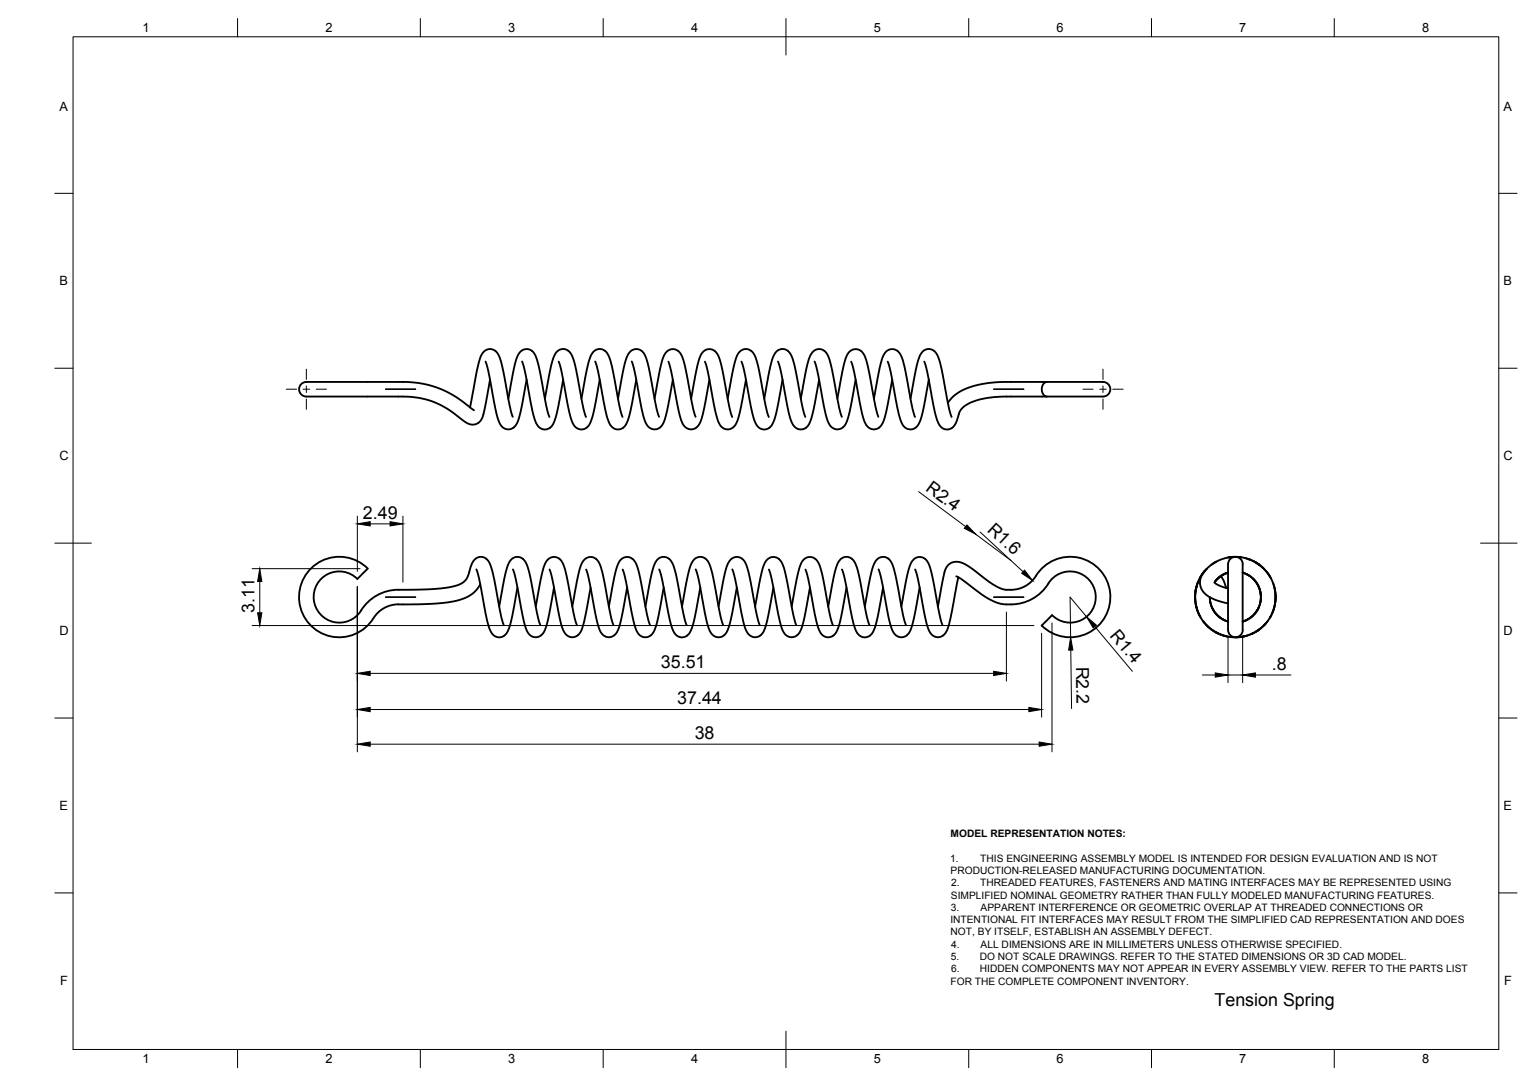
ISO-10303-21;
HEADER;
/* Generated by software containing ST-Developer
 * from STEP Tools, Inc. (www.steptools.com) 
 */

FILE_DESCRIPTION(
/* description */ ('STEP AP214'),
/* implementation_level */ '2;1');

FILE_NAME(
/* name */ 'Tension Spring.step',
/* time_stamp */ '2026-10-06T11:11:25-07:00',
/* author */ (''),
/* organization */ (''),
/* preprocessor_version */ 'ST-DEVELOPER v20.2',
/* originating_system */ 'Autodesk Translation Framework v15.15.0.0',
/* authorisation */ '');

FILE_SCHEMA (('AUTOMOTIVE_DESIGN { 1 0 10303 214 3 1 1 }'));
ENDSEC;

DATA;
#10=MECHANICAL_DESIGN_GEOMETRIC_PRESENTATION_REPRESENTATION('',(#699),#47717);
#148=B_SPLINE_CURVE_WITH_KNOTS('',3,(#12437,#12438,#12439,#12440,#12441,
#12442,#12443,#12444,#12445,#12446,#12447,#12448,#12449,#12450,#12451,#12452,
#12453,#12454,#12455,#12456,#12457,#12458,#12459,#12460),.UNSPECIFIED.,
 .F.,.F.,(4,2,2,2,2,2,2,2,2,2,2,4),(0.916063809045508,0.917441355582055,
0.918818902118601,0.921573995191693,0.924329088264786,0.925706634801332,
0.927084181337879,0.932594367484064,0.935349460557156,0.936727007093702,
0.937415780361976,0.938104553630249),.UNSPECIFIED.);
#149=B_SPLINE_CURVE_WITH_KNOTS('',3,(#12461,#12462,#12463,#12464,#12465,
#12466,#12467,#12468,#12469,#12470,#12471,#12472,#12473,#12474,#12475,#12476,
#12477,#12478,#12479,#12480,#12481,#12482,#12483,#12484),.UNSPECIFIED.,
 .F.,.F.,(4,2,2,2,2,2,2,2,2,2,2,4),(0.916063809045508,0.917441355582055,
0.918818902118601,0.921573995191693,0.924329088264786,0.925706634801332,
0.927084181337879,0.932594367484064,0.935349460557156,0.936727007093702,
0.937415780361976,0.938104553630249),.UNSPECIFIED.);
#150=B_SPLINE_CURVE_WITH_KNOTS('',3,(#13664,#13665,#13666,#13667,#13668,
#13669,#13670,#13671,#13672,#13673,#13674,#13675,#13676,#13677,#13678,#13679,
#13680,#13681,#13682,#13683,#13684,#13685,#13686,#13687,#13688,#13689,#13690,
#13691,#13692,#13693,#13694,#13695,#13696,#13697,#13698,#13699,#13700,#13701,
#13702,#13703,#13704,#13705,#13706,#13707,#13708,#13709,#13710,#13711,#13712,
#13713,#13714,#13715,#13716,#13717,#13718,#13719,#13720,#13721,#13722,#13723,
#13724,#13725,#13726,#13727,#13728,#13729,#13730,#13731,#13732,#13733,#13734,
#13735,#13736,#13737,#13738,#13739,#13740,#13741,#13742,#13743,#13744,#13745,
#13746,#13747,#13748,#13749,#13750,#13751,#13752,#13753,#13754,#13755,#13756,
#13757,#13758,#13759,#13760,#13761,#13762,#13763,#13764,#13765,#13766,#13767,
#13768,#13769,#13770,#13771,#13772,#13773,#13774,#13775,#13776,#13777,#13778,
#13779,#13780,#13781,#13782,#13783,#13784,#13785,#13786,#13787,#13788,#13789,
#13790,#13791,#13792,#13793,#13794,#13795,#13796,#13797,#13798,#13799,#13800,
#13801,#13802,#13803,#13804,#13805,#13806,#13807,#13808,#13809,#13810,#13811,
#13812,#13813,#13814,#13815,#13816,#13817,#13818,#13819,#13820,#13821,#13822,
#13823,#13824,#13825,#13826,#13827,#13828,#13829,#13830,#13831),
 .UNSPECIFIED.,.F.,.F.,(4,2,2,2,2,2,2,2,2,2,2,2,2,2,2,2,2,2,2,2,2,2,2,2,
2,2,2,2,2,2,2,2,2,2,2,2,2,2,2,2,2,2,2,2,2,2,2,2,2,2,2,2,2,2,2,2,2,2,2,2,
2,2,2,2,2,2,2,2,2,2,2,2,2,2,2,2,2,2,2,2,2,2,2,4),(0.0896131586159842,0.0909349273058256,
0.092256695995667,0.09490023337535,0.100187308134716,0.110761457653447,
0.121335607172179,0.131909756690911,0.142406945548381,0.152904134405852,
0.163401323263323,0.173898512120793,0.184326267064866,0.194754022008939,
0.205181776953011,0.215609531897084,0.225968774255778,0.236328016614473,
0.246687258973167,0.257046501331861,0.268365392558388,0.279684283784914,
0.29100317501144,0.302322066237966,0.313563979866736,0.324805893495506,
0.336047807124276,0.347289720753047,0.358457560536344,0.369625400319641,
0.380793240102939,0.391961079886236,0.403057648451734,0.414154217017233,
0.425250785582731,0.43634735414823,0.447375242283774,0.458403130419317,
0.469431018554861,0.480458906690405,0.491420626849432,0.50238234700846,
0.513344067167488,0.524305787326516,0.535203741266554,0.546101695206592,
0.55699964914663,0.567897603086667,0.578734005374906,0.589570407663145,
0.600406809951383,0.611243212239622,0.62202044333232,0.632797674425018,
0.643574905517716,0.654352136610414,0.665072195325672,0.675792254040929,
0.686512312756186,0.697232371471444,0.707897173370898,0.718561975270352,
0.729226777169807,0.739891579069261,0.750503305564763,0.761115032060264,
0.771726758555766,0.782338485051268,0.79289871583597,0.803458946620673,
0.814019177405375,0.824579408190078,0.835090233536042,0.845601058882007,
0.856111884227971,0.866622709573936,0.877085607262584,0.887548504951232,
0.89801140263988,0.908474300328528,0.912269054687018,0.914166431866263,
0.915115120455886,0.916063809045508),.UNSPECIFIED.);
#151=B_SPLINE_CURVE_WITH_KNOTS('',3,(#13832,#13833,#13834,#13835,#13836,
#13837,#13838,#13839,#13840,#13841,#13842,#13843,#13844,#13845,#13846,#13847,
#13848,#13849,#13850,#13851,#13852,#13853,#13854,#13855,#13856,#13857,#13858,
#13859,#13860,#13861,#13862,#13863,#13864,#13865,#13866,#13867,#13868,#13869,
#13870,#13871,#13872,#13873,#13874,#13875,#13876,#13877,#13878,#13879,#13880,
#13881,#13882,#13883,#13884,#13885,#13886,#13887,#13888,#13889,#13890,#13891,
#13892,#13893,#13894,#13895,#13896,#13897,#13898,#13899,#13900,#13901,#13902,
#13903,#13904,#13905,#13906,#13907,#13908,#13909,#13910,#13911,#13912,#13913,
#13914,#13915,#13916,#13917,#13918,#13919,#13920,#13921,#13922,#13923,#13924,
#13925,#13926,#13927,#13928,#13929,#13930,#13931,#13932,#13933,#13934,#13935,
#13936,#13937,#13938,#13939,#13940,#13941,#13942,#13943,#13944,#13945,#13946,
#13947,#13948,#13949,#13950,#13951,#13952,#13953,#13954,#13955,#13956,#13957,
#13958,#13959,#13960,#13961,#13962,#13963,#13964,#13965,#13966,#13967,#13968,
#13969,#13970,#13971,#13972,#13973,#13974,#13975,#13976,#13977,#13978,#13979,
#13980,#13981,#13982,#13983,#13984,#13985,#13986,#13987,#13988,#13989,#13990,
#13991,#13992,#13993,#13994,#13995,#13996,#13997,#13998,#13999),
 .UNSPECIFIED.,.F.,.F.,(4,2,2,2,2,2,2,2,2,2,2,2,2,2,2,2,2,2,2,2,2,2,2,2,
2,2,2,2,2,2,2,2,2,2,2,2,2,2,2,2,2,2,2,2,2,2,2,2,2,2,2,2,2,2,2,2,2,2,2,2,
2,2,2,2,2,2,2,2,2,2,2,2,2,2,2,2,2,2,2,2,2,2,2,4),(0.0896131586159842,0.0909349273058256,
0.092256695995667,0.09490023337535,0.100187308134716,0.110761457653447,
0.121335607172179,0.131909756690911,0.142406945548381,0.152904134405852,
0.163401323263323,0.173898512120793,0.184326267064866,0.194754022008939,
0.205181776953011,0.215609531897084,0.225968774255778,0.236328016614473,
0.246687258973167,0.257046501331861,0.268365392558388,0.279684283784914,
0.29100317501144,0.302322066237966,0.313563979866736,0.324805893495506,
0.336047807124276,0.347289720753047,0.358457560536344,0.369625400319641,
0.380793240102939,0.391961079886236,0.403057648451734,0.414154217017233,
0.425250785582731,0.43634735414823,0.447375242283774,0.458403130419317,
0.469431018554861,0.480458906690405,0.491420626849432,0.50238234700846,
0.513344067167488,0.524305787326516,0.535203741266554,0.546101695206592,
0.55699964914663,0.567897603086667,0.578734005374906,0.589570407663145,
0.600406809951383,0.611243212239622,0.62202044333232,0.632797674425018,
0.643574905517716,0.654352136610414,0.665072195325672,0.675792254040929,
0.686512312756186,0.697232371471444,0.707897173370898,0.718561975270352,
0.729226777169807,0.739891579069261,0.750503305564763,0.761115032060264,
0.771726758555766,0.782338485051268,0.79289871583597,0.803458946620673,
0.814019177405375,0.824579408190078,0.835090233536042,0.845601058882007,
0.856111884227971,0.866622709573936,0.877085607262584,0.887548504951232,
0.89801140263988,0.908474300328528,0.912269054687018,0.914166431866263,
0.915115120455886,0.916063809045508),.UNSPECIFIED.);
#152=B_SPLINE_CURVE_WITH_KNOTS('',3,(#14143,#14144,#14145,#14146,#14147,
#14148,#14149,#14150,#14151,#14152,#14153,#14154,#14155,#14156,#14157,#14158,
#14159,#14160,#14161,#14162),.UNSPECIFIED.,.F.,.F.,(4,2,2,2,2,2,2,2,2,4),
(0.0618954463697512,0.0653601604005303,0.0688248744313094,0.0757543024928677,
0.0792190165236468,0.0809513735390363,0.0826837305544259,0.086148444585205,
0.0878808016005946,0.0896131586159842),.UNSPECIFIED.);
#153=B_SPLINE_CURVE_WITH_KNOTS('',3,(#14163,#14164,#14165,#14166,#14167,
#14168,#14169,#14170,#14171,#14172,#14173,#14174,#14175,#14176,#14177,#14178,
#14179,#14180,#14181,#14182),.UNSPECIFIED.,.F.,.F.,(4,2,2,2,2,2,2,2,2,4),
(0.0618954463697512,0.0653601604005303,0.0688248744313094,0.0757543024928677,
0.0792190165236468,0.0809513735390363,0.0826837305544259,0.086148444585205,
0.0878808016005946,0.0896131586159842),.UNSPECIFIED.);
#526=(
BOUNDED_SURFACE()
B_SPLINE_SURFACE(3,3,((#12266,#12267,#12268,#12269,#12270,#12271,#12272,
#12273,#12274,#12275,#12276,#12277,#12278,#12279,#12280,#12281,#12282,#12283,
#12284,#12285,#12286,#12287,#12288,#12289),(#12290,#12291,#12292,#12293,
#12294,#12295,#12296,#12297,#12298,#12299,#12300,#12301,#12302,#12303,#12304,
#12305,#12306,#12307,#12308,#12309,#12310,#12311,#12312,#12313),(#12314,
#12315,#12316,#12317,#12318,#12319,#12320,#12321,#12322,#12323,#12324,#12325,
#12326,#12327,#12328,#12329,#12330,#12331,#12332,#12333,#12334,#12335,#12336,
#12337),(#12338,#12339,#12340,#12341,#12342,#12343,#12344,#12345,#12346,
#12347,#12348,#12349,#12350,#12351,#12352,#12353,#12354,#12355,#12356,#12357,
#12358,#12359,#12360,#12361),(#12362,#12363,#12364,#12365,#12366,#12367,
#12368,#12369,#12370,#12371,#12372,#12373,#12374,#12375,#12376,#12377,#12378,
#12379,#12380,#12381,#12382,#12383,#12384,#12385),(#12386,#12387,#12388,
#12389,#12390,#12391,#12392,#12393,#12394,#12395,#12396,#12397,#12398,#12399,
#12400,#12401,#12402,#12403,#12404,#12405,#12406,#12407,#12408,#12409),
(#12410,#12411,#12412,#12413,#12414,#12415,#12416,#12417,#12418,#12419,
#12420,#12421,#12422,#12423,#12424,#12425,#12426,#12427,#12428,#12429,#12430,
#12431,#12432,#12433)),.UNSPECIFIED.,.T.,.F.,.F.)
B_SPLINE_SURFACE_WITH_KNOTS((4,3,4),(4,2,2,2,2,2,2,2,2,2,2,4),(0.,0.5,1.),
(0.916063809045508,0.917441355582055,0.918818902118601,0.921573995191693,
0.924329088264786,0.925706634801332,0.927084181337879,0.932594367484064,
0.935349460557156,0.936727007093702,0.937415780361976,0.938104553630249),
 .UNSPECIFIED.)
GEOMETRIC_REPRESENTATION_ITEM()
RATIONAL_B_SPLINE_SURFACE(((1.,1.,1.,1.,1.,1.,1.,1.,1.,1.,1.,1.,1.,1.,1.,
1.,1.,1.,1.,1.,1.,1.,1.,1.),(0.333333333333333,0.333333333333333,0.333333333333333,
0.333333333333333,0.333333333333333,0.333333333333333,0.333333333333333,
0.333333333333333,0.333333333333333,0.333333333333333,0.333333333333333,
0.333333333333333,0.333333333333333,0.333333333333333,0.333333333333333,
0.333333333333333,0.333333333333333,0.333333333333333,0.333333333333333,
0.333333333333333,0.333333333333333,0.333333333333333,0.333333333333333,
0.333333333333333),(0.333333333333333,0.333333333333333,0.333333333333333,
0.333333333333333,0.333333333333333,0.333333333333333,0.333333333333333,
0.333333333333333,0.333333333333333,0.333333333333333,0.333333333333333,
0.333333333333333,0.333333333333333,0.333333333333333,0.333333333333333,
0.333333333333333,0.333333333333333,0.333333333333333,0.333333333333333,
0.333333333333333,0.333333333333333,0.333333333333333,0.333333333333333,
0.333333333333333),(1.,1.,1.,1.,1.,1.,1.,1.,1.,1.,1.,1.,1.,1.,1.,1.,1.,
1.,1.,1.,1.,1.,1.,1.),(0.333333333333333,0.333333333333333,0.333333333333333,
0.333333333333333,0.333333333333333,0.333333333333333,0.333333333333333,
0.333333333333333,0.333333333333333,0.333333333333333,0.333333333333333,
0.333333333333333,0.333333333333333,0.333333333333333,0.333333333333333,
0.333333333333333,0.333333333333333,0.333333333333333,0.333333333333333,
0.333333333333333,0.333333333333333,0.333333333333333,0.333333333333333,
0.333333333333333),(0.333333333333333,0.333333333333333,0.333333333333333,
0.333333333333333,0.333333333333333,0.333333333333333,0.333333333333333,
0.333333333333333,0.333333333333333,0.333333333333333,0.333333333333333,
0.333333333333333,0.333333333333333,0.333333333333333,0.333333333333333,
0.333333333333333,0.333333333333333,0.333333333333333,0.333333333333333,
0.333333333333333,0.333333333333333,0.333333333333333,0.333333333333333,
0.333333333333333),(1.,1.,1.,1.,1.,1.,1.,1.,1.,1.,1.,1.,1.,1.,1.,1.,1.,
1.,1.,1.,1.,1.,1.,1.)))
REPRESENTATION_ITEM('')
SURFACE()
);
#527=(
BOUNDED_SURFACE()
B_SPLINE_SURFACE(3,3,((#12485,#12486,#12487,#12488,#12489,#12490,#12491,
#12492,#12493,#12494,#12495,#12496,#12497,#12498,#12499,#12500,#12501,#12502,
#12503,#12504,#12505,#12506,#12507,#12508,#12509,#12510,#12511,#12512,#12513,
#12514,#12515,#12516,#12517,#12518,#12519,#12520,#12521,#12522,#12523,#12524,
#12525,#12526,#12527,#12528,#12529,#12530,#12531,#12532,#12533,#12534,#12535,
#12536,#12537,#12538,#12539,#12540,#12541,#12542,#12543,#12544,#12545,#12546,
#12547,#12548,#12549,#12550,#12551,#12552,#12553,#12554,#12555,#12556,#12557,
#12558,#12559,#12560,#12561,#12562,#12563,#12564,#12565,#12566,#12567,#12568,
#12569,#12570,#12571,#12572,#12573,#12574,#12575,#12576,#12577,#12578,#12579,
#12580,#12581,#12582,#12583,#12584,#12585,#12586,#12587,#12588,#12589,#12590,
#12591,#12592,#12593,#12594,#12595,#12596,#12597,#12598,#12599,#12600,#12601,
#12602,#12603,#12604,#12605,#12606,#12607,#12608,#12609,#12610,#12611,#12612,
#12613,#12614,#12615,#12616,#12617,#12618,#12619,#12620,#12621,#12622,#12623,
#12624,#12625,#12626,#12627,#12628,#12629,#12630,#12631,#12632,#12633,#12634,
#12635,#12636,#12637,#12638,#12639,#12640,#12641,#12642,#12643,#12644,#12645,
#12646,#12647,#12648,#12649,#12650,#12651,#12652),(#12653,#12654,#12655,
#12656,#12657,#12658,#12659,#12660,#12661,#12662,#12663,#12664,#12665,#12666,
#12667,#12668,#12669,#12670,#12671,#12672,#12673,#12674,#12675,#12676,#12677,
#12678,#12679,#12680,#12681,#12682,#12683,#12684,#12685,#12686,#12687,#12688,
#12689,#12690,#12691,#12692,#12693,#12694,#12695,#12696,#12697,#12698,#12699,
#12700,#12701,#12702,#12703,#12704,#12705,#12706,#12707,#12708,#12709,#12710,
#12711,#12712,#12713,#12714,#12715,#12716,#12717,#12718,#12719,#12720,#12721,
#12722,#12723,#12724,#12725,#12726,#12727,#12728,#12729,#12730,#12731,#12732,
#12733,#12734,#12735,#12736,#12737,#12738,#12739,#12740,#12741,#12742,#12743,
#12744,#12745,#12746,#12747,#12748,#12749,#12750,#12751,#12752,#12753,#12754,
#12755,#12756,#12757,#12758,#12759,#12760,#12761,#12762,#12763,#12764,#12765,
#12766,#12767,#12768,#12769,#12770,#12771,#12772,#12773,#12774,#12775,#12776,
#12777,#12778,#12779,#12780,#12781,#12782,#12783,#12784,#12785,#12786,#12787,
#12788,#12789,#12790,#12791,#12792,#12793,#12794,#12795,#12796,#12797,#12798,
#12799,#12800,#12801,#12802,#12803,#12804,#12805,#12806,#12807,#12808,#12809,
#12810,#12811,#12812,#12813,#12814,#12815,#12816,#12817,#12818,#12819,#12820),
(#12821,#12822,#12823,#12824,#12825,#12826,#12827,#12828,#12829,#12830,
#12831,#12832,#12833,#12834,#12835,#12836,#12837,#12838,#12839,#12840,#12841,
#12842,#12843,#12844,#12845,#12846,#12847,#12848,#12849,#12850,#12851,#12852,
#12853,#12854,#12855,#12856,#12857,#12858,#12859,#12860,#12861,#12862,#12863,
#12864,#12865,#12866,#12867,#12868,#12869,#12870,#12871,#12872,#12873,#12874,
#12875,#12876,#12877,#12878,#12879,#12880,#12881,#12882,#12883,#12884,#12885,
#12886,#12887,#12888,#12889,#12890,#12891,#12892,#12893,#12894,#12895,#12896,
#12897,#12898,#12899,#12900,#12901,#12902,#12903,#12904,#12905,#12906,#12907,
#12908,#12909,#12910,#12911,#12912,#12913,#12914,#12915,#12916,#12917,#12918,
#12919,#12920,#12921,#12922,#12923,#12924,#12925,#12926,#12927,#12928,#12929,
#12930,#12931,#12932,#12933,#12934,#12935,#12936,#12937,#12938,#12939,#12940,
#12941,#12942,#12943,#12944,#12945,#12946,#12947,#12948,#12949,#12950,#12951,
#12952,#12953,#12954,#12955,#12956,#12957,#12958,#12959,#12960,#12961,#12962,
#12963,#12964,#12965,#12966,#12967,#12968,#12969,#12970,#12971,#12972,#12973,
#12974,#12975,#12976,#12977,#12978,#12979,#12980,#12981,#12982,#12983,#12984,
#12985,#12986,#12987,#12988),(#12989,#12990,#12991,#12992,#12993,#12994,
#12995,#12996,#12997,#12998,#12999,#13000,#13001,#13002,#13003,#13004,#13005,
#13006,#13007,#13008,#13009,#13010,#13011,#13012,#13013,#13014,#13015,#13016,
#13017,#13018,#13019,#13020,#13021,#13022,#13023,#13024,#13025,#13026,#13027,
#13028,#13029,#13030,#13031,#13032,#13033,#13034,#13035,#13036,#13037,#13038,
#13039,#13040,#13041,#13042,#13043,#13044,#13045,#13046,#13047,#13048,#13049,
#13050,#13051,#13052,#13053,#13054,#13055,#13056,#13057,#13058,#13059,#13060,
#13061,#13062,#13063,#13064,#13065,#13066,#13067,#13068,#13069,#13070,#13071,
#13072,#13073,#13074,#13075,#13076,#13077,#13078,#13079,#13080,#13081,#13082,
#13083,#13084,#13085,#13086,#13087,#13088,#13089,#13090,#13091,#13092,#13093,
#13094,#13095,#13096,#13097,#13098,#13099,#13100,#13101,#13102,#13103,#13104,
#13105,#13106,#13107,#13108,#13109,#13110,#13111,#13112,#13113,#13114,#13115,
#13116,#13117,#13118,#13119,#13120,#13121,#13122,#13123,#13124,#13125,#13126,
#13127,#13128,#13129,#13130,#13131,#13132,#13133,#13134,#13135,#13136,#13137,
#13138,#13139,#13140,#13141,#13142,#13143,#13144,#13145,#13146,#13147,#13148,
#13149,#13150,#13151,#13152,#13153,#13154,#13155,#13156),(#13157,#13158,
#13159,#13160,#13161,#13162,#13163,#13164,#13165,#13166,#13167,#13168,#13169,
#13170,#13171,#13172,#13173,#13174,#13175,#13176,#13177,#13178,#13179,#13180,
#13181,#13182,#13183,#13184,#13185,#13186,#13187,#13188,#13189,#13190,#13191,
#13192,#13193,#13194,#13195,#13196,#13197,#13198,#13199,#13200,#13201,#13202,
#13203,#13204,#13205,#13206,#13207,#13208,#13209,#13210,#13211,#13212,#13213,
#13214,#13215,#13216,#13217,#13218,#13219,#13220,#13221,#13222,#13223,#13224,
#13225,#13226,#13227,#13228,#13229,#13230,#13231,#13232,#13233,#13234,#13235,
#13236,#13237,#13238,#13239,#13240,#13241,#13242,#13243,#13244,#13245,#13246,
#13247,#13248,#13249,#13250,#13251,#13252,#13253,#13254,#13255,#13256,#13257,
#13258,#13259,#13260,#13261,#13262,#13263,#13264,#13265,#13266,#13267,#13268,
#13269,#13270,#13271,#13272,#13273,#13274,#13275,#13276,#13277,#13278,#13279,
#13280,#13281,#13282,#13283,#13284,#13285,#13286,#13287,#13288,#13289,#13290,
#13291,#13292,#13293,#13294,#13295,#13296,#13297,#13298,#13299,#13300,#13301,
#13302,#13303,#13304,#13305,#13306,#13307,#13308,#13309,#13310,#13311,#13312,
#13313,#13314,#13315,#13316,#13317,#13318,#13319,#13320,#13321,#13322,#13323,
#13324),(#13325,#13326,#13327,#13328,#13329,#13330,#13331,#13332,#13333,
#13334,#13335,#13336,#13337,#13338,#13339,#13340,#13341,#13342,#13343,#13344,
#13345,#13346,#13347,#13348,#13349,#13350,#13351,#13352,#13353,#13354,#13355,
#13356,#13357,#13358,#13359,#13360,#13361,#13362,#13363,#13364,#13365,#13366,
#13367,#13368,#13369,#13370,#13371,#13372,#13373,#13374,#13375,#13376,#13377,
#13378,#13379,#13380,#13381,#13382,#13383,#13384,#13385,#13386,#13387,#13388,
#13389,#13390,#13391,#13392,#13393,#13394,#13395,#13396,#13397,#13398,#13399,
#13400,#13401,#13402,#13403,#13404,#13405,#13406,#13407,#13408,#13409,#13410,
#13411,#13412,#13413,#13414,#13415,#13416,#13417,#13418,#13419,#13420,#13421,
#13422,#13423,#13424,#13425,#13426,#13427,#13428,#13429,#13430,#13431,#13432,
#13433,#13434,#13435,#13436,#13437,#13438,#13439,#13440,#13441,#13442,#13443,
#13444,#13445,#13446,#13447,#13448,#13449,#13450,#13451,#13452,#13453,#13454,
#13455,#13456,#13457,#13458,#13459,#13460,#13461,#13462,#13463,#13464,#13465,
#13466,#13467,#13468,#13469,#13470,#13471,#13472,#13473,#13474,#13475,#13476,
#13477,#13478,#13479,#13480,#13481,#13482,#13483,#13484,#13485,#13486,#13487,
#13488,#13489,#13490,#13491,#13492),(#13493,#13494,#13495,#13496,#13497,
#13498,#13499,#13500,#13501,#13502,#13503,#13504,#13505,#13506,#13507,#13508,
#13509,#13510,#13511,#13512,#13513,#13514,#13515,#13516,#13517,#13518,#13519,
#13520,#13521,#13522,#13523,#13524,#13525,#13526,#13527,#13528,#13529,#13530,
#13531,#13532,#13533,#13534,#13535,#13536,#13537,#13538,#13539,#13540,#13541,
#13542,#13543,#13544,#13545,#13546,#13547,#13548,#13549,#13550,#13551,#13552,
#13553,#13554,#13555,#13556,#13557,#13558,#13559,#13560,#13561,#13562,#13563,
#13564,#13565,#13566,#13567,#13568,#13569,#13570,#13571,#13572,#13573,#13574,
#13575,#13576,#13577,#13578,#13579,#13580,#13581,#13582,#13583,#13584,#13585,
#13586,#13587,#13588,#13589,#13590,#13591,#13592,#13593,#13594,#13595,#13596,
#13597,#13598,#13599,#13600,#13601,#13602,#13603,#13604,#13605,#13606,#13607,
#13608,#13609,#13610,#13611,#13612,#13613,#13614,#13615,#13616,#13617,#13618,
#13619,#13620,#13621,#13622,#13623,#13624,#13625,#13626,#13627,#13628,#13629,
#13630,#13631,#13632,#13633,#13634,#13635,#13636,#13637,#13638,#13639,#13640,
#13641,#13642,#13643,#13644,#13645,#13646,#13647,#13648,#13649,#13650,#13651,
#13652,#13653,#13654,#13655,#13656,#13657,#13658,#13659,#13660)),
 .UNSPECIFIED.,.T.,.F.,.F.)
B_SPLINE_SURFACE_WITH_KNOTS((4,3,4),(4,2,2,2,2,2,2,2,2,2,2,2,2,2,2,2,2,
2,2,2,2,2,2,2,2,2,2,2,2,2,2,2,2,2,2,2,2,2,2,2,2,2,2,2,2,2,2,2,2,2,2,2,2,
2,2,2,2,2,2,2,2,2,2,2,2,2,2,2,2,2,2,2,2,2,2,2,2,2,2,2,2,2,2,4),(0.,0.5,
1.),(0.0896131586159842,0.0909349273058256,0.092256695995667,0.09490023337535,
0.100187308134716,0.110761457653447,0.121335607172179,0.131909756690911,
0.142406945548381,0.152904134405852,0.163401323263323,0.173898512120793,
0.184326267064866,0.194754022008939,0.205181776953011,0.215609531897084,
0.225968774255778,0.236328016614473,0.246687258973167,0.257046501331861,
0.268365392558388,0.279684283784914,0.29100317501144,0.302322066237966,
0.313563979866736,0.324805893495506,0.336047807124276,0.347289720753047,
0.358457560536344,0.369625400319641,0.380793240102939,0.391961079886236,
0.403057648451734,0.414154217017233,0.425250785582731,0.43634735414823,
0.447375242283774,0.458403130419317,0.469431018554861,0.480458906690405,
0.491420626849432,0.50238234700846,0.513344067167488,0.524305787326516,
0.535203741266554,0.546101695206592,0.55699964914663,0.567897603086667,
0.578734005374906,0.589570407663145,0.600406809951383,0.611243212239622,
0.62202044333232,0.632797674425018,0.643574905517716,0.654352136610414,
0.665072195325672,0.675792254040929,0.686512312756186,0.697232371471444,
0.707897173370898,0.718561975270352,0.729226777169807,0.739891579069261,
0.750503305564763,0.761115032060264,0.771726758555766,0.782338485051267,
0.79289871583597,0.803458946620673,0.814019177405375,0.824579408190078,
0.835090233536042,0.845601058882007,0.856111884227971,0.866622709573936,
0.877085607262584,0.887548504951232,0.89801140263988,0.908474300328528,
0.912269054687018,0.914166431866263,0.915115120455886,0.916063809045508),
 .UNSPECIFIED.)
GEOMETRIC_REPRESENTATION_ITEM()
RATIONAL_B_SPLINE_SURFACE(((1.,1.,1.,1.,1.,1.,1.,1.,1.,1.,1.,1.,1.,1.,1.,
1.,1.,1.,1.,1.,1.,1.,1.,1.,1.,1.,1.,1.,1.,1.,1.,1.,1.,1.,1.,1.,1.,1.,1.,
1.,1.,1.,1.,1.,1.,1.,1.,1.,1.,1.,1.,1.,1.,1.,1.,1.,1.,1.,1.,1.,1.,1.,1.,
1.,1.,1.,1.,1.,1.,1.,1.,1.,1.,1.,1.,1.,1.,1.,1.,1.,1.,1.,1.,1.,1.,1.,1.,
1.,1.,1.,1.,1.,1.,1.,1.,1.,1.,1.,1.,1.,1.,1.,1.,1.,1.,1.,1.,1.,1.,1.,1.,
1.,1.,1.,1.,1.,1.,1.,1.,1.,1.,1.,1.,1.,1.,1.,1.,1.,1.,1.,1.,1.,1.,1.,1.,
1.,1.,1.,1.,1.,1.,1.,1.,1.,1.,1.,1.,1.,1.,1.,1.,1.,1.,1.,1.,1.,1.,1.,1.,
1.,1.,1.,1.,1.,1.,1.,1.,1.),(0.333333333333333,0.333333333333333,0.333333333333333,
0.333333333333333,0.333333333333333,0.333333333333333,0.333333333333333,
0.333333333333333,0.333333333333333,0.333333333333333,0.333333333333333,
0.333333333333333,0.333333333333333,0.333333333333333,0.333333333333333,
0.333333333333333,0.333333333333333,0.333333333333333,0.333333333333333,
0.333333333333333,0.333333333333333,0.333333333333333,0.333333333333333,
0.333333333333333,0.333333333333333,0.333333333333333,0.333333333333333,
0.333333333333333,0.333333333333333,0.333333333333333,0.333333333333333,
0.333333333333333,0.333333333333333,0.333333333333333,0.333333333333333,
0.333333333333333,0.333333333333333,0.333333333333333,0.333333333333333,
0.333333333333333,0.333333333333333,0.333333333333333,0.333333333333333,
0.333333333333333,0.333333333333333,0.333333333333333,0.333333333333333,
0.333333333333333,0.333333333333333,0.333333333333333,0.333333333333333,
0.333333333333333,0.333333333333333,0.333333333333333,0.333333333333333,
0.333333333333333,0.333333333333333,0.333333333333333,0.333333333333333,
0.333333333333333,0.333333333333333,0.333333333333333,0.333333333333333,
0.333333333333333,0.333333333333333,0.333333333333333,0.333333333333333,
0.333333333333333,0.333333333333333,0.333333333333333,0.333333333333333,
0.333333333333333,0.333333333333333,0.333333333333333,0.333333333333333,
0.333333333333333,0.333333333333333,0.333333333333333,0.333333333333333,
0.333333333333333,0.333333333333333,0.333333333333333,0.333333333333333,
0.333333333333333,0.333333333333333,0.333333333333333,0.333333333333333,
0.333333333333333,0.333333333333333,0.333333333333333,0.333333333333333,
0.333333333333333,0.333333333333333,0.333333333333333,0.333333333333333,
0.333333333333333,0.333333333333333,0.333333333333333,0.333333333333333,
0.333333333333333,0.333333333333333,0.333333333333333,0.333333333333333,
0.333333333333333,0.333333333333333,0.333333333333333,0.333333333333333,
0.333333333333333,0.333333333333333,0.333333333333333,0.333333333333333,
0.333333333333333,0.333333333333333,0.333333333333333,0.333333333333333,
0.333333333333333,0.333333333333333,0.333333333333333,0.333333333333333,
0.333333333333333,0.333333333333333,0.333333333333333,0.333333333333333,
0.333333333333333,0.333333333333333,0.333333333333333,0.333333333333333,
0.333333333333333,0.333333333333333,0.333333333333333,0.333333333333333,
0.333333333333333,0.333333333333333,0.333333333333333,0.333333333333333,
0.333333333333333,0.333333333333333,0.333333333333333,0.333333333333333,
0.333333333333333,0.333333333333333,0.333333333333333,0.333333333333333,
0.333333333333333,0.333333333333333,0.333333333333333,0.333333333333333,
0.333333333333333,0.333333333333333,0.333333333333333,0.333333333333333,
0.333333333333333,0.333333333333333,0.333333333333333,0.333333333333333,
0.333333333333333,0.333333333333333,0.333333333333333,0.333333333333333,
0.333333333333333,0.333333333333333,0.333333333333333,0.333333333333333,
0.333333333333333,0.333333333333333,0.333333333333333,0.333333333333333,
0.333333333333333),(0.333333333333333,0.333333333333333,0.333333333333333,
0.333333333333333,0.333333333333333,0.333333333333333,0.333333333333333,
0.333333333333333,0.333333333333333,0.333333333333333,0.333333333333333,
0.333333333333333,0.333333333333333,0.333333333333333,0.333333333333333,
0.333333333333333,0.333333333333333,0.333333333333333,0.333333333333333,
0.333333333333333,0.333333333333333,0.333333333333333,0.333333333333333,
0.333333333333333,0.333333333333333,0.333333333333333,0.333333333333333,
0.333333333333333,0.333333333333333,0.333333333333333,0.333333333333333,
0.333333333333333,0.333333333333333,0.333333333333333,0.333333333333333,
0.333333333333333,0.333333333333333,0.333333333333333,0.333333333333333,
0.333333333333333,0.333333333333333,0.333333333333333,0.333333333333333,
0.333333333333333,0.333333333333333,0.333333333333333,0.333333333333333,
0.333333333333333,0.333333333333333,0.333333333333333,0.333333333333333,
0.333333333333333,0.333333333333333,0.333333333333333,0.333333333333333,
0.333333333333333,0.333333333333333,0.333333333333333,0.333333333333333,
0.333333333333333,0.333333333333333,0.333333333333333,0.333333333333333,
0.333333333333333,0.333333333333333,0.333333333333333,0.333333333333333,
0.333333333333333,0.333333333333333,0.333333333333333,0.333333333333333,
0.333333333333333,0.333333333333333,0.333333333333333,0.333333333333333,
0.333333333333333,0.333333333333333,0.333333333333333,0.333333333333333,
0.333333333333333,0.333333333333333,0.333333333333333,0.333333333333333,
0.333333333333333,0.333333333333333,0.333333333333333,0.333333333333333,
0.333333333333333,0.333333333333333,0.333333333333333,0.333333333333333,
0.333333333333333,0.333333333333333,0.333333333333333,0.333333333333333,
0.333333333333333,0.333333333333333,0.333333333333333,0.333333333333333,
0.333333333333333,0.333333333333333,0.333333333333333,0.333333333333333,
0.333333333333333,0.333333333333333,0.333333333333333,0.333333333333333,
0.333333333333333,0.333333333333333,0.333333333333333,0.333333333333333,
0.333333333333333,0.333333333333333,0.333333333333333,0.333333333333333,
0.333333333333333,0.333333333333333,0.333333333333333,0.333333333333333,
0.333333333333333,0.333333333333333,0.333333333333333,0.333333333333333,
0.333333333333333,0.333333333333333,0.333333333333333,0.333333333333333,
0.333333333333333,0.333333333333333,0.333333333333333,0.333333333333333,
0.333333333333333,0.333333333333333,0.333333333333333,0.333333333333333,
0.333333333333333,0.333333333333333,0.333333333333333,0.333333333333333,
0.333333333333333,0.333333333333333,0.333333333333333,0.333333333333333,
0.333333333333333,0.333333333333333,0.333333333333333,0.333333333333333,
0.333333333333333,0.333333333333333,0.333333333333333,0.333333333333333,
0.333333333333333,0.333333333333333,0.333333333333333,0.333333333333333,
0.333333333333333,0.333333333333333,0.333333333333333,0.333333333333333,
0.333333333333333,0.333333333333333,0.333333333333333,0.333333333333333,
0.333333333333333,0.333333333333333,0.333333333333333,0.333333333333333,
0.333333333333333),(1.,1.,1.,1.,1.,1.,1.,1.,1.,1.,1.,1.,1.,1.,1.,1.,1.,
1.,1.,1.,1.,1.,1.,1.,1.,1.,1.,1.,1.,1.,1.,1.,1.,1.,1.,1.,1.,1.,1.,1.,1.,
1.,1.,1.,1.,1.,1.,1.,1.,1.,1.,1.,1.,1.,1.,1.,1.,1.,1.,1.,1.,1.,1.,1.,1.,
1.,1.,1.,1.,1.,1.,1.,1.,1.,1.,1.,1.,1.,1.,1.,1.,1.,1.,1.,1.,1.,1.,1.,1.,
1.,1.,1.,1.,1.,1.,1.,1.,1.,1.,1.,1.,1.,1.,1.,1.,1.,1.,1.,1.,1.,1.,1.,1.,
1.,1.,1.,1.,1.,1.,1.,1.,1.,1.,1.,1.,1.,1.,1.,1.,1.,1.,1.,1.,1.,1.,1.,1.,
1.,1.,1.,1.,1.,1.,1.,1.,1.,1.,1.,1.,1.,1.,1.,1.,1.,1.,1.,1.,1.,1.,1.,1.,
1.,1.,1.,1.,1.,1.,1.),(0.333333333333333,0.333333333333333,0.333333333333333,
0.333333333333333,0.333333333333333,0.333333333333333,0.333333333333333,
0.333333333333333,0.333333333333333,0.333333333333333,0.333333333333333,
0.333333333333333,0.333333333333333,0.333333333333333,0.333333333333333,
0.333333333333333,0.333333333333333,0.333333333333333,0.333333333333333,
0.333333333333333,0.333333333333333,0.333333333333333,0.333333333333333,
0.333333333333333,0.333333333333333,0.333333333333333,0.333333333333333,
0.333333333333333,0.333333333333333,0.333333333333333,0.333333333333333,
0.333333333333333,0.333333333333333,0.333333333333333,0.333333333333333,
0.333333333333333,0.333333333333333,0.333333333333333,0.333333333333333,
0.333333333333333,0.333333333333333,0.333333333333333,0.333333333333333,
0.333333333333333,0.333333333333333,0.333333333333333,0.333333333333333,
0.333333333333333,0.333333333333333,0.333333333333333,0.333333333333333,
0.333333333333333,0.333333333333333,0.333333333333333,0.333333333333333,
0.333333333333333,0.333333333333333,0.333333333333333,0.333333333333333,
0.333333333333333,0.333333333333333,0.333333333333333,0.333333333333333,
0.333333333333333,0.333333333333333,0.333333333333333,0.333333333333333,
0.333333333333333,0.333333333333333,0.333333333333333,0.333333333333333,
0.333333333333333,0.333333333333333,0.333333333333333,0.333333333333333,
0.333333333333333,0.333333333333333,0.333333333333333,0.333333333333333,
0.333333333333333,0.333333333333333,0.333333333333333,0.333333333333333,
0.333333333333333,0.333333333333333,0.333333333333333,0.333333333333333,
0.333333333333333,0.333333333333333,0.333333333333333,0.333333333333333,
0.333333333333333,0.333333333333333,0.333333333333333,0.333333333333333,
0.333333333333333,0.333333333333333,0.333333333333333,0.333333333333333,
0.333333333333333,0.333333333333333,0.333333333333333,0.333333333333333,
0.333333333333333,0.333333333333333,0.333333333333333,0.333333333333333,
0.333333333333333,0.333333333333333,0.333333333333333,0.333333333333333,
0.333333333333333,0.333333333333333,0.333333333333333,0.333333333333333,
0.333333333333333,0.333333333333333,0.333333333333333,0.333333333333333,
0.333333333333333,0.333333333333333,0.333333333333333,0.333333333333333,
0.333333333333333,0.333333333333333,0.333333333333333,0.333333333333333,
0.333333333333333,0.333333333333333,0.333333333333333,0.333333333333333,
0.333333333333333,0.333333333333333,0.333333333333333,0.333333333333333,
0.333333333333333,0.333333333333333,0.333333333333333,0.333333333333333,
0.333333333333333,0.333333333333333,0.333333333333333,0.333333333333333,
0.333333333333333,0.333333333333333,0.333333333333333,0.333333333333333,
0.333333333333333,0.333333333333333,0.333333333333333,0.333333333333333,
0.333333333333333,0.333333333333333,0.333333333333333,0.333333333333333,
0.333333333333333,0.333333333333333,0.333333333333333,0.333333333333333,
0.333333333333333,0.333333333333333,0.333333333333333,0.333333333333333,
0.333333333333333,0.333333333333333,0.333333333333333,0.333333333333333,
0.333333333333333),(0.333333333333333,0.333333333333333,0.333333333333333,
0.333333333333333,0.333333333333333,0.333333333333333,0.333333333333333,
0.333333333333333,0.333333333333333,0.333333333333333,0.333333333333333,
0.333333333333333,0.333333333333333,0.333333333333333,0.333333333333333,
0.333333333333333,0.333333333333333,0.333333333333333,0.333333333333333,
0.333333333333333,0.333333333333333,0.333333333333333,0.333333333333333,
0.333333333333333,0.333333333333333,0.333333333333333,0.333333333333333,
0.333333333333333,0.333333333333333,0.333333333333333,0.333333333333333,
0.333333333333333,0.333333333333333,0.333333333333333,0.333333333333333,
0.333333333333333,0.333333333333333,0.333333333333333,0.333333333333333,
0.333333333333333,0.333333333333333,0.333333333333333,0.333333333333333,
0.333333333333333,0.333333333333333,0.333333333333333,0.333333333333333,
0.333333333333333,0.333333333333333,0.333333333333333,0.333333333333333,
0.333333333333333,0.333333333333333,0.333333333333333,0.333333333333333,
0.333333333333333,0.333333333333333,0.333333333333333,0.333333333333333,
0.333333333333333,0.333333333333333,0.333333333333333,0.333333333333333,
0.333333333333333,0.333333333333333,0.333333333333333,0.333333333333333,
0.333333333333333,0.333333333333333,0.333333333333333,0.333333333333333,
0.333333333333333,0.333333333333333,0.333333333333333,0.333333333333333,
0.333333333333333,0.333333333333333,0.333333333333333,0.333333333333333,
0.333333333333333,0.333333333333333,0.333333333333333,0.333333333333333,
0.333333333333333,0.333333333333333,0.333333333333333,0.333333333333333,
0.333333333333333,0.333333333333333,0.333333333333333,0.333333333333333,
0.333333333333333,0.333333333333333,0.333333333333333,0.333333333333333,
0.333333333333333,0.333333333333333,0.333333333333333,0.333333333333333,
0.333333333333333,0.333333333333333,0.333333333333333,0.333333333333333,
0.333333333333333,0.333333333333333,0.333333333333333,0.333333333333333,
0.333333333333333,0.333333333333333,0.333333333333333,0.333333333333333,
0.333333333333333,0.333333333333333,0.333333333333333,0.333333333333333,
0.333333333333333,0.333333333333333,0.333333333333333,0.333333333333333,
0.333333333333333,0.333333333333333,0.333333333333333,0.333333333333333,
0.333333333333333,0.333333333333333,0.333333333333333,0.333333333333333,
0.333333333333333,0.333333333333333,0.333333333333333,0.333333333333333,
0.333333333333333,0.333333333333333,0.333333333333333,0.333333333333333,
0.333333333333333,0.333333333333333,0.333333333333333,0.333333333333333,
0.333333333333333,0.333333333333333,0.333333333333333,0.333333333333333,
0.333333333333333,0.333333333333333,0.333333333333333,0.333333333333333,
0.333333333333333,0.333333333333333,0.333333333333333,0.333333333333333,
0.333333333333333,0.333333333333333,0.333333333333333,0.333333333333333,
0.333333333333333,0.333333333333333,0.333333333333333,0.333333333333333,
0.333333333333333,0.333333333333333,0.333333333333333,0.333333333333333,
0.333333333333333,0.333333333333333,0.333333333333333,0.333333333333333,
0.333333333333333),(1.,1.,1.,1.,1.,1.,1.,1.,1.,1.,1.,1.,1.,1.,1.,1.,1.,
1.,1.,1.,1.,1.,1.,1.,1.,1.,1.,1.,1.,1.,1.,1.,1.,1.,1.,1.,1.,1.,1.,1.,1.,
1.,1.,1.,1.,1.,1.,1.,1.,1.,1.,1.,1.,1.,1.,1.,1.,1.,1.,1.,1.,1.,1.,1.,1.,
1.,1.,1.,1.,1.,1.,1.,1.,1.,1.,1.,1.,1.,1.,1.,1.,1.,1.,1.,1.,1.,1.,1.,1.,
1.,1.,1.,1.,1.,1.,1.,1.,1.,1.,1.,1.,1.,1.,1.,1.,1.,1.,1.,1.,1.,1.,1.,1.,
1.,1.,1.,1.,1.,1.,1.,1.,1.,1.,1.,1.,1.,1.,1.,1.,1.,1.,1.,1.,1.,1.,1.,1.,
1.,1.,1.,1.,1.,1.,1.,1.,1.,1.,1.,1.,1.,1.,1.,1.,1.,1.,1.,1.,1.,1.,1.,1.,
1.,1.,1.,1.,1.,1.,1.)))
REPRESENTATION_ITEM('')
SURFACE()
);
#528=(
BOUNDED_SURFACE()
B_SPLINE_SURFACE(3,3,((#14000,#14001,#14002,#14003,#14004,#14005,#14006,
#14007,#14008,#14009,#14010,#14011,#14012,#14013,#14014,#14015,#14016,#14017,
#14018,#14019),(#14020,#14021,#14022,#14023,#14024,#14025,#14026,#14027,
#14028,#14029,#14030,#14031,#14032,#14033,#14034,#14035,#14036,#14037,#14038,
#14039),(#14040,#14041,#14042,#14043,#14044,#14045,#14046,#14047,#14048,
#14049,#14050,#14051,#14052,#14053,#14054,#14055,#14056,#14057,#14058,#14059),
(#14060,#14061,#14062,#14063,#14064,#14065,#14066,#14067,#14068,#14069,
#14070,#14071,#14072,#14073,#14074,#14075,#14076,#14077,#14078,#14079),
(#14080,#14081,#14082,#14083,#14084,#14085,#14086,#14087,#14088,#14089,
#14090,#14091,#14092,#14093,#14094,#14095,#14096,#14097,#14098,#14099),
(#14100,#14101,#14102,#14103,#14104,#14105,#14106,#14107,#14108,#14109,
#14110,#14111,#14112,#14113,#14114,#14115,#14116,#14117,#14118,#14119),
(#14120,#14121,#14122,#14123,#14124,#14125,#14126,#14127,#14128,#14129,
#14130,#14131,#14132,#14133,#14134,#14135,#14136,#14137,#14138,#14139)),
 .UNSPECIFIED.,.T.,.F.,.F.)
B_SPLINE_SURFACE_WITH_KNOTS((4,3,4),(4,2,2,2,2,2,2,2,2,4),(0.,0.5,1.),(0.0618954463697512,
0.0653601604005303,0.0688248744313094,0.0757543024928677,0.0792190165236468,
0.0809513735390363,0.0826837305544259,0.086148444585205,0.0878808016005946,
0.0896131586159842),.UNSPECIFIED.)
GEOMETRIC_REPRESENTATION_ITEM()
RATIONAL_B_SPLINE_SURFACE(((1.,1.,1.,1.,1.,1.,1.,1.,1.,1.,1.,1.,1.,1.,1.,
1.,1.,1.,1.,1.),(0.333333333333333,0.333333333333333,0.333333333333333,
0.333333333333333,0.333333333333333,0.333333333333333,0.333333333333333,
0.333333333333333,0.333333333333333,0.333333333333333,0.333333333333333,
0.333333333333333,0.333333333333333,0.333333333333333,0.333333333333333,
0.333333333333333,0.333333333333333,0.333333333333333,0.333333333333333,
0.333333333333333),(0.333333333333333,0.333333333333333,0.333333333333333,
0.333333333333333,0.333333333333333,0.333333333333333,0.333333333333333,
0.333333333333333,0.333333333333333,0.333333333333333,0.333333333333333,
0.333333333333333,0.333333333333333,0.333333333333333,0.333333333333333,
0.333333333333333,0.333333333333333,0.333333333333333,0.333333333333333,
0.333333333333333),(1.,1.,1.,1.,1.,1.,1.,1.,1.,1.,1.,1.,1.,1.,1.,1.,1.,
1.,1.,1.),(0.333333333333333,0.333333333333333,0.333333333333333,0.333333333333333,
0.333333333333333,0.333333333333333,0.333333333333333,0.333333333333333,
0.333333333333333,0.333333333333333,0.333333333333333,0.333333333333333,
0.333333333333333,0.333333333333333,0.333333333333333,0.333333333333333,
0.333333333333333,0.333333333333333,0.333333333333333,0.333333333333333),
(0.333333333333333,0.333333333333333,0.333333333333333,0.333333333333333,
0.333333333333333,0.333333333333333,0.333333333333333,0.333333333333333,
0.333333333333333,0.333333333333333,0.333333333333333,0.333333333333333,
0.333333333333333,0.333333333333333,0.333333333333333,0.333333333333333,
0.333333333333333,0.333333333333333,0.333333333333333,0.333333333333333),
(1.,1.,1.,1.,1.,1.,1.,1.,1.,1.,1.,1.,1.,1.,1.,1.,1.,1.,1.,1.)))
REPRESENTATION_ITEM('')
SURFACE()
);
#529=(
BOUNDED_SURFACE()
B_SPLINE_SURFACE(3,3,((#14186,#14187,#14188,#14189,#14190,#14191,#14192,
#14193,#14194,#14195,#14196,#14197,#14198,#14199,#14200,#14201,#14202,#14203,
#14204,#14205,#14206,#14207,#14208,#14209),(#14210,#14211,#14212,#14213,
#14214,#14215,#14216,#14217,#14218,#14219,#14220,#14221,#14222,#14223,#14224,
#14225,#14226,#14227,#14228,#14229,#14230,#14231,#14232,#14233),(#14234,
#14235,#14236,#14237,#14238,#14239,#14240,#14241,#14242,#14243,#14244,#14245,
#14246,#14247,#14248,#14249,#14250,#14251,#14252,#14253,#14254,#14255,#14256,
#14257),(#14258,#14259,#14260,#14261,#14262,#14263,#14264,#14265,#14266,
#14267,#14268,#14269,#14270,#14271,#14272,#14273,#14274,#14275,#14276,#14277,
#14278,#14279,#14280,#14281),(#14282,#14283,#14284,#14285,#14286,#14287,
#14288,#14289,#14290,#14291,#14292,#14293,#14294,#14295,#14296,#14297,#14298,
#14299,#14300,#14301,#14302,#14303,#14304,#14305),(#14306,#14307,#14308,
#14309,#14310,#14311,#14312,#14313,#14314,#14315,#14316,#14317,#14318,#14319,
#14320,#14321,#14322,#14323,#14324,#14325,#14326,#14327,#14328,#14329),
(#14330,#14331,#14332,#14333,#14334,#14335,#14336,#14337,#14338,#14339,
#14340,#14341,#14342,#14343,#14344,#14345,#14346,#14347,#14348,#14349,#14350,
#14351,#14352,#14353)),.UNSPECIFIED.,.T.,.F.,.F.)
B_SPLINE_SURFACE_WITH_KNOTS((4,3,4),(4,2,2,2,2,2,2,2,2,2,2,4),(0.,0.5,1.),
(0.916063809045508,0.917441355582055,0.918818902118601,0.921573995191693,
0.924329088264786,0.925706634801332,0.927084181337879,0.932594367484064,
0.935349460557156,0.936727007093702,0.937415780361976,0.938104553630249),
 .UNSPECIFIED.)
GEOMETRIC_REPRESENTATION_ITEM()
RATIONAL_B_SPLINE_SURFACE(((1.,1.,1.,1.,1.,1.,1.,1.,1.,1.,1.,1.,1.,1.,1.,
1.,1.,1.,1.,1.,1.,1.,1.,1.),(0.333333333333333,0.333333333333333,0.333333333333333,
0.333333333333333,0.333333333333333,0.333333333333333,0.333333333333333,
0.333333333333333,0.333333333333333,0.333333333333333,0.333333333333333,
0.333333333333333,0.333333333333333,0.333333333333333,0.333333333333333,
0.333333333333333,0.333333333333333,0.333333333333333,0.333333333333333,
0.333333333333333,0.333333333333333,0.333333333333333,0.333333333333333,
0.333333333333333),(0.333333333333333,0.333333333333333,0.333333333333333,
0.333333333333333,0.333333333333333,0.333333333333333,0.333333333333333,
0.333333333333333,0.333333333333333,0.333333333333333,0.333333333333333,
0.333333333333333,0.333333333333333,0.333333333333333,0.333333333333333,
0.333333333333333,0.333333333333333,0.333333333333333,0.333333333333333,
0.333333333333333,0.333333333333333,0.333333333333333,0.333333333333333,
0.333333333333333),(1.,1.,1.,1.,1.,1.,1.,1.,1.,1.,1.,1.,1.,1.,1.,1.,1.,
1.,1.,1.,1.,1.,1.,1.),(0.333333333333333,0.333333333333333,0.333333333333333,
0.333333333333333,0.333333333333333,0.333333333333333,0.333333333333333,
0.333333333333333,0.333333333333333,0.333333333333333,0.333333333333333,
0.333333333333333,0.333333333333333,0.333333333333333,0.333333333333333,
0.333333333333333,0.333333333333333,0.333333333333333,0.333333333333333,
0.333333333333333,0.333333333333333,0.333333333333333,0.333333333333333,
0.333333333333333),(0.333333333333333,0.333333333333333,0.333333333333333,
0.333333333333333,0.333333333333333,0.333333333333333,0.333333333333333,
0.333333333333333,0.333333333333333,0.333333333333333,0.333333333333333,
0.333333333333333,0.333333333333333,0.333333333333333,0.333333333333333,
0.333333333333333,0.333333333333333,0.333333333333333,0.333333333333333,
0.333333333333333,0.333333333333333,0.333333333333333,0.333333333333333,
0.333333333333333),(1.,1.,1.,1.,1.,1.,1.,1.,1.,1.,1.,1.,1.,1.,1.,1.,1.,
1.,1.,1.,1.,1.,1.,1.)))
REPRESENTATION_ITEM('')
SURFACE()
);
#530=(
BOUNDED_SURFACE()
B_SPLINE_SURFACE(3,3,((#14355,#14356,#14357,#14358,#14359,#14360,#14361,
#14362,#14363,#14364,#14365,#14366,#14367,#14368,#14369,#14370,#14371,#14372,
#14373,#14374,#14375,#14376,#14377,#14378,#14379,#14380,#14381,#14382,#14383,
#14384,#14385,#14386,#14387,#14388,#14389,#14390,#14391,#14392,#14393,#14394,
#14395,#14396,#14397,#14398,#14399,#14400,#14401,#14402,#14403,#14404,#14405,
#14406,#14407,#14408,#14409,#14410,#14411,#14412,#14413,#14414,#14415,#14416,
#14417,#14418,#14419,#14420,#14421,#14422,#14423,#14424,#14425,#14426,#14427,
#14428,#14429,#14430,#14431,#14432,#14433,#14434,#14435,#14436,#14437,#14438,
#14439,#14440,#14441,#14442,#14443,#14444,#14445,#14446,#14447,#14448,#14449,
#14450,#14451,#14452,#14453,#14454,#14455,#14456,#14457,#14458,#14459,#14460,
#14461,#14462,#14463,#14464,#14465,#14466,#14467,#14468,#14469,#14470,#14471,
#14472,#14473,#14474,#14475,#14476,#14477,#14478,#14479,#14480,#14481,#14482,
#14483,#14484,#14485,#14486,#14487,#14488,#14489,#14490,#14491,#14492,#14493,
#14494,#14495,#14496,#14497,#14498,#14499,#14500,#14501,#14502,#14503,#14504,
#14505,#14506,#14507,#14508,#14509,#14510,#14511,#14512,#14513,#14514,#14515,
#14516,#14517,#14518,#14519,#14520,#14521,#14522),(#14523,#14524,#14525,
#14526,#14527,#14528,#14529,#14530,#14531,#14532,#14533,#14534,#14535,#14536,
#14537,#14538,#14539,#14540,#14541,#14542,#14543,#14544,#14545,#14546,#14547,
#14548,#14549,#14550,#14551,#14552,#14553,#14554,#14555,#14556,#14557,#14558,
#14559,#14560,#14561,#14562,#14563,#14564,#14565,#14566,#14567,#14568,#14569,
#14570,#14571,#14572,#14573,#14574,#14575,#14576,#14577,#14578,#14579,#14580,
#14581,#14582,#14583,#14584,#14585,#14586,#14587,#14588,#14589,#14590,#14591,
#14592,#14593,#14594,#14595,#14596,#14597,#14598,#14599,#14600,#14601,#14602,
#14603,#14604,#14605,#14606,#14607,#14608,#14609,#14610,#14611,#14612,#14613,
#14614,#14615,#14616,#14617,#14618,#14619,#14620,#14621,#14622,#14623,#14624,
#14625,#14626,#14627,#14628,#14629,#14630,#14631,#14632,#14633,#14634,#14635,
#14636,#14637,#14638,#14639,#14640,#14641,#14642,#14643,#14644,#14645,#14646,
#14647,#14648,#14649,#14650,#14651,#14652,#14653,#14654,#14655,#14656,#14657,
#14658,#14659,#14660,#14661,#14662,#14663,#14664,#14665,#14666,#14667,#14668,
#14669,#14670,#14671,#14672,#14673,#14674,#14675,#14676,#14677,#14678,#14679,
#14680,#14681,#14682,#14683,#14684,#14685,#14686,#14687,#14688,#14689,#14690),
(#14691,#14692,#14693,#14694,#14695,#14696,#14697,#14698,#14699,#14700,
#14701,#14702,#14703,#14704,#14705,#14706,#14707,#14708,#14709,#14710,#14711,
#14712,#14713,#14714,#14715,#14716,#14717,#14718,#14719,#14720,#14721,#14722,
#14723,#14724,#14725,#14726,#14727,#14728,#14729,#14730,#14731,#14732,#14733,
#14734,#14735,#14736,#14737,#14738,#14739,#14740,#14741,#14742,#14743,#14744,
#14745,#14746,#14747,#14748,#14749,#14750,#14751,#14752,#14753,#14754,#14755,
#14756,#14757,#14758,#14759,#14760,#14761,#14762,#14763,#14764,#14765,#14766,
#14767,#14768,#14769,#14770,#14771,#14772,#14773,#14774,#14775,#14776,#14777,
#14778,#14779,#14780,#14781,#14782,#14783,#14784,#14785,#14786,#14787,#14788,
#14789,#14790,#14791,#14792,#14793,#14794,#14795,#14796,#14797,#14798,#14799,
#14800,#14801,#14802,#14803,#14804,#14805,#14806,#14807,#14808,#14809,#14810,
#14811,#14812,#14813,#14814,#14815,#14816,#14817,#14818,#14819,#14820,#14821,
#14822,#14823,#14824,#14825,#14826,#14827,#14828,#14829,#14830,#14831,#14832,
#14833,#14834,#14835,#14836,#14837,#14838,#14839,#14840,#14841,#14842,#14843,
#14844,#14845,#14846,#14847,#14848,#14849,#14850,#14851,#14852,#14853,#14854,
#14855,#14856,#14857,#14858),(#14859,#14860,#14861,#14862,#14863,#14864,
#14865,#14866,#14867,#14868,#14869,#14870,#14871,#14872,#14873,#14874,#14875,
#14876,#14877,#14878,#14879,#14880,#14881,#14882,#14883,#14884,#14885,#14886,
#14887,#14888,#14889,#14890,#14891,#14892,#14893,#14894,#14895,#14896,#14897,
#14898,#14899,#14900,#14901,#14902,#14903,#14904,#14905,#14906,#14907,#14908,
#14909,#14910,#14911,#14912,#14913,#14914,#14915,#14916,#14917,#14918,#14919,
#14920,#14921,#14922,#14923,#14924,#14925,#14926,#14927,#14928,#14929,#14930,
#14931,#14932,#14933,#14934,#14935,#14936,#14937,#14938,#14939,#14940,#14941,
#14942,#14943,#14944,#14945,#14946,#14947,#14948,#14949,#14950,#14951,#14952,
#14953,#14954,#14955,#14956,#14957,#14958,#14959,#14960,#14961,#14962,#14963,
#14964,#14965,#14966,#14967,#14968,#14969,#14970,#14971,#14972,#14973,#14974,
#14975,#14976,#14977,#14978,#14979,#14980,#14981,#14982,#14983,#14984,#14985,
#14986,#14987,#14988,#14989,#14990,#14991,#14992,#14993,#14994,#14995,#14996,
#14997,#14998,#14999,#15000,#15001,#15002,#15003,#15004,#15005,#15006,#15007,
#15008,#15009,#15010,#15011,#15012,#15013,#15014,#15015,#15016,#15017,#15018,
#15019,#15020,#15021,#15022,#15023,#15024,#15025,#15026),(#15027,#15028,
#15029,#15030,#15031,#15032,#15033,#15034,#15035,#15036,#15037,#15038,#15039,
#15040,#15041,#15042,#15043,#15044,#15045,#15046,#15047,#15048,#15049,#15050,
#15051,#15052,#15053,#15054,#15055,#15056,#15057,#15058,#15059,#15060,#15061,
#15062,#15063,#15064,#15065,#15066,#15067,#15068,#15069,#15070,#15071,#15072,
#15073,#15074,#15075,#15076,#15077,#15078,#15079,#15080,#15081,#15082,#15083,
#15084,#15085,#15086,#15087,#15088,#15089,#15090,#15091,#15092,#15093,#15094,
#15095,#15096,#15097,#15098,#15099,#15100,#15101,#15102,#15103,#15104,#15105,
#15106,#15107,#15108,#15109,#15110,#15111,#15112,#15113,#15114,#15115,#15116,
#15117,#15118,#15119,#15120,#15121,#15122,#15123,#15124,#15125,#15126,#15127,
#15128,#15129,#15130,#15131,#15132,#15133,#15134,#15135,#15136,#15137,#15138,
#15139,#15140,#15141,#15142,#15143,#15144,#15145,#15146,#15147,#15148,#15149,
#15150,#15151,#15152,#15153,#15154,#15155,#15156,#15157,#15158,#15159,#15160,
#15161,#15162,#15163,#15164,#15165,#15166,#15167,#15168,#15169,#15170,#15171,
#15172,#15173,#15174,#15175,#15176,#15177,#15178,#15179,#15180,#15181,#15182,
#15183,#15184,#15185,#15186,#15187,#15188,#15189,#15190,#15191,#15192,#15193,
#15194),(#15195,#15196,#15197,#15198,#15199,#15200,#15201,#15202,#15203,
#15204,#15205,#15206,#15207,#15208,#15209,#15210,#15211,#15212,#15213,#15214,
#15215,#15216,#15217,#15218,#15219,#15220,#15221,#15222,#15223,#15224,#15225,
#15226,#15227,#15228,#15229,#15230,#15231,#15232,#15233,#15234,#15235,#15236,
#15237,#15238,#15239,#15240,#15241,#15242,#15243,#15244,#15245,#15246,#15247,
#15248,#15249,#15250,#15251,#15252,#15253,#15254,#15255,#15256,#15257,#15258,
#15259,#15260,#15261,#15262,#15263,#15264,#15265,#15266,#15267,#15268,#15269,
#15270,#15271,#15272,#15273,#15274,#15275,#15276,#15277,#15278,#15279,#15280,
#15281,#15282,#15283,#15284,#15285,#15286,#15287,#15288,#15289,#15290,#15291,
#15292,#15293,#15294,#15295,#15296,#15297,#15298,#15299,#15300,#15301,#15302,
#15303,#15304,#15305,#15306,#15307,#15308,#15309,#15310,#15311,#15312,#15313,
#15314,#15315,#15316,#15317,#15318,#15319,#15320,#15321,#15322,#15323,#15324,
#15325,#15326,#15327,#15328,#15329,#15330,#15331,#15332,#15333,#15334,#15335,
#15336,#15337,#15338,#15339,#15340,#15341,#15342,#15343,#15344,#15345,#15346,
#15347,#15348,#15349,#15350,#15351,#15352,#15353,#15354,#15355,#15356,#15357,
#15358,#15359,#15360,#15361,#15362),(#15363,#15364,#15365,#15366,#15367,
#15368,#15369,#15370,#15371,#15372,#15373,#15374,#15375,#15376,#15377,#15378,
#15379,#15380,#15381,#15382,#15383,#15384,#15385,#15386,#15387,#15388,#15389,
#15390,#15391,#15392,#15393,#15394,#15395,#15396,#15397,#15398,#15399,#15400,
#15401,#15402,#15403,#15404,#15405,#15406,#15407,#15408,#15409,#15410,#15411,
#15412,#15413,#15414,#15415,#15416,#15417,#15418,#15419,#15420,#15421,#15422,
#15423,#15424,#15425,#15426,#15427,#15428,#15429,#15430,#15431,#15432,#15433,
#15434,#15435,#15436,#15437,#15438,#15439,#15440,#15441,#15442,#15443,#15444,
#15445,#15446,#15447,#15448,#15449,#15450,#15451,#15452,#15453,#15454,#15455,
#15456,#15457,#15458,#15459,#15460,#15461,#15462,#15463,#15464,#15465,#15466,
#15467,#15468,#15469,#15470,#15471,#15472,#15473,#15474,#15475,#15476,#15477,
#15478,#15479,#15480,#15481,#15482,#15483,#15484,#15485,#15486,#15487,#15488,
#15489,#15490,#15491,#15492,#15493,#15494,#15495,#15496,#15497,#15498,#15499,
#15500,#15501,#15502,#15503,#15504,#15505,#15506,#15507,#15508,#15509,#15510,
#15511,#15512,#15513,#15514,#15515,#15516,#15517,#15518,#15519,#15520,#15521,
#15522,#15523,#15524,#15525,#15526,#15527,#15528,#15529,#15530)),
 .UNSPECIFIED.,.T.,.F.,.F.)
B_SPLINE_SURFACE_WITH_KNOTS((4,3,4),(4,2,2,2,2,2,2,2,2,2,2,2,2,2,2,2,2,
2,2,2,2,2,2,2,2,2,2,2,2,2,2,2,2,2,2,2,2,2,2,2,2,2,2,2,2,2,2,2,2,2,2,2,2,
2,2,2,2,2,2,2,2,2,2,2,2,2,2,2,2,2,2,2,2,2,2,2,2,2,2,2,2,2,2,4),(0.,0.5,
1.),(0.0896131586159842,0.0909349273058256,0.092256695995667,0.09490023337535,
0.100187308134716,0.110761457653447,0.121335607172179,0.131909756690911,
0.142406945548381,0.152904134405852,0.163401323263323,0.173898512120793,
0.184326267064866,0.194754022008939,0.205181776953011,0.215609531897084,
0.225968774255778,0.236328016614473,0.246687258973167,0.257046501331861,
0.268365392558388,0.279684283784914,0.29100317501144,0.302322066237966,
0.313563979866736,0.324805893495506,0.336047807124276,0.347289720753047,
0.358457560536344,0.369625400319641,0.380793240102939,0.391961079886236,
0.403057648451734,0.414154217017233,0.425250785582731,0.43634735414823,
0.447375242283774,0.458403130419317,0.469431018554861,0.480458906690405,
0.491420626849432,0.50238234700846,0.513344067167488,0.524305787326516,
0.535203741266554,0.546101695206592,0.55699964914663,0.567897603086667,
0.578734005374906,0.589570407663145,0.600406809951383,0.611243212239622,
0.62202044333232,0.632797674425018,0.643574905517716,0.654352136610414,
0.665072195325672,0.675792254040929,0.686512312756186,0.697232371471444,
0.707897173370898,0.718561975270352,0.729226777169807,0.739891579069261,
0.750503305564763,0.761115032060264,0.771726758555766,0.782338485051267,
0.79289871583597,0.803458946620673,0.814019177405375,0.824579408190078,
0.835090233536042,0.845601058882007,0.856111884227971,0.866622709573936,
0.877085607262584,0.887548504951232,0.89801140263988,0.908474300328528,
0.912269054687018,0.914166431866263,0.915115120455886,0.916063809045508),
 .UNSPECIFIED.)
GEOMETRIC_REPRESENTATION_ITEM()
RATIONAL_B_SPLINE_SURFACE(((1.,1.,1.,1.,1.,1.,1.,1.,1.,1.,1.,1.,1.,1.,1.,
1.,1.,1.,1.,1.,1.,1.,1.,1.,1.,1.,1.,1.,1.,1.,1.,1.,1.,1.,1.,1.,1.,1.,1.,
1.,1.,1.,1.,1.,1.,1.,1.,1.,1.,1.,1.,1.,1.,1.,1.,1.,1.,1.,1.,1.,1.,1.,1.,
1.,1.,1.,1.,1.,1.,1.,1.,1.,1.,1.,1.,1.,1.,1.,1.,1.,1.,1.,1.,1.,1.,1.,1.,
1.,1.,1.,1.,1.,1.,1.,1.,1.,1.,1.,1.,1.,1.,1.,1.,1.,1.,1.,1.,1.,1.,1.,1.,
1.,1.,1.,1.,1.,1.,1.,1.,1.,1.,1.,1.,1.,1.,1.,1.,1.,1.,1.,1.,1.,1.,1.,1.,
1.,1.,1.,1.,1.,1.,1.,1.,1.,1.,1.,1.,1.,1.,1.,1.,1.,1.,1.,1.,1.,1.,1.,1.,
1.,1.,1.,1.,1.,1.,1.,1.,1.),(0.333333333333333,0.333333333333333,0.333333333333333,
0.333333333333333,0.333333333333333,0.333333333333333,0.333333333333333,
0.333333333333333,0.333333333333333,0.333333333333333,0.333333333333333,
0.333333333333333,0.333333333333333,0.333333333333333,0.333333333333333,
0.333333333333333,0.333333333333333,0.333333333333333,0.333333333333333,
0.333333333333333,0.333333333333333,0.333333333333333,0.333333333333333,
0.333333333333333,0.333333333333333,0.333333333333333,0.333333333333333,
0.333333333333333,0.333333333333333,0.333333333333333,0.333333333333333,
0.333333333333333,0.333333333333333,0.333333333333333,0.333333333333333,
0.333333333333333,0.333333333333333,0.333333333333333,0.333333333333333,
0.333333333333333,0.333333333333333,0.333333333333333,0.333333333333333,
0.333333333333333,0.333333333333333,0.333333333333333,0.333333333333333,
0.333333333333333,0.333333333333333,0.333333333333333,0.333333333333333,
0.333333333333333,0.333333333333333,0.333333333333333,0.333333333333333,
0.333333333333333,0.333333333333333,0.333333333333333,0.333333333333333,
0.333333333333333,0.333333333333333,0.333333333333333,0.333333333333333,
0.333333333333333,0.333333333333333,0.333333333333333,0.333333333333333,
0.333333333333333,0.333333333333333,0.333333333333333,0.333333333333333,
0.333333333333333,0.333333333333333,0.333333333333333,0.333333333333333,
0.333333333333333,0.333333333333333,0.333333333333333,0.333333333333333,
0.333333333333333,0.333333333333333,0.333333333333333,0.333333333333333,
0.333333333333333,0.333333333333333,0.333333333333333,0.333333333333333,
0.333333333333333,0.333333333333333,0.333333333333333,0.333333333333333,
0.333333333333333,0.333333333333333,0.333333333333333,0.333333333333333,
0.333333333333333,0.333333333333333,0.333333333333333,0.333333333333333,
0.333333333333333,0.333333333333333,0.333333333333333,0.333333333333333,
0.333333333333333,0.333333333333333,0.333333333333333,0.333333333333333,
0.333333333333333,0.333333333333333,0.333333333333333,0.333333333333333,
0.333333333333333,0.333333333333333,0.333333333333333,0.333333333333333,
0.333333333333333,0.333333333333333,0.333333333333333,0.333333333333333,
0.333333333333333,0.333333333333333,0.333333333333333,0.333333333333333,
0.333333333333333,0.333333333333333,0.333333333333333,0.333333333333333,
0.333333333333333,0.333333333333333,0.333333333333333,0.333333333333333,
0.333333333333333,0.333333333333333,0.333333333333333,0.333333333333333,
0.333333333333333,0.333333333333333,0.333333333333333,0.333333333333333,
0.333333333333333,0.333333333333333,0.333333333333333,0.333333333333333,
0.333333333333333,0.333333333333333,0.333333333333333,0.333333333333333,
0.333333333333333,0.333333333333333,0.333333333333333,0.333333333333333,
0.333333333333333,0.333333333333333,0.333333333333333,0.333333333333333,
0.333333333333333,0.333333333333333,0.333333333333333,0.333333333333333,
0.333333333333333,0.333333333333333,0.333333333333333,0.333333333333333,
0.333333333333333,0.333333333333333,0.333333333333333,0.333333333333333,
0.333333333333333),(0.333333333333333,0.333333333333333,0.333333333333333,
0.333333333333333,0.333333333333333,0.333333333333333,0.333333333333333,
0.333333333333333,0.333333333333333,0.333333333333333,0.333333333333333,
0.333333333333333,0.333333333333333,0.333333333333333,0.333333333333333,
0.333333333333333,0.333333333333333,0.333333333333333,0.333333333333333,
0.333333333333333,0.333333333333333,0.333333333333333,0.333333333333333,
0.333333333333333,0.333333333333333,0.333333333333333,0.333333333333333,
0.333333333333333,0.333333333333333,0.333333333333333,0.333333333333333,
0.333333333333333,0.333333333333333,0.333333333333333,0.333333333333333,
0.333333333333333,0.333333333333333,0.333333333333333,0.333333333333333,
0.333333333333333,0.333333333333333,0.333333333333333,0.333333333333333,
0.333333333333333,0.333333333333333,0.333333333333333,0.333333333333333,
0.333333333333333,0.333333333333333,0.333333333333333,0.333333333333333,
0.333333333333333,0.333333333333333,0.333333333333333,0.333333333333333,
0.333333333333333,0.333333333333333,0.333333333333333,0.333333333333333,
0.333333333333333,0.333333333333333,0.333333333333333,0.333333333333333,
0.333333333333333,0.333333333333333,0.333333333333333,0.333333333333333,
0.333333333333333,0.333333333333333,0.333333333333333,0.333333333333333,
0.333333333333333,0.333333333333333,0.333333333333333,0.333333333333333,
0.333333333333333,0.333333333333333,0.333333333333333,0.333333333333333,
0.333333333333333,0.333333333333333,0.333333333333333,0.333333333333333,
0.333333333333333,0.333333333333333,0.333333333333333,0.333333333333333,
0.333333333333333,0.333333333333333,0.333333333333333,0.333333333333333,
0.333333333333333,0.333333333333333,0.333333333333333,0.333333333333333,
0.333333333333333,0.333333333333333,0.333333333333333,0.333333333333333,
0.333333333333333,0.333333333333333,0.333333333333333,0.333333333333333,
0.333333333333333,0.333333333333333,0.333333333333333,0.333333333333333,
0.333333333333333,0.333333333333333,0.333333333333333,0.333333333333333,
0.333333333333333,0.333333333333333,0.333333333333333,0.333333333333333,
0.333333333333333,0.333333333333333,0.333333333333333,0.333333333333333,
0.333333333333333,0.333333333333333,0.333333333333333,0.333333333333333,
0.333333333333333,0.333333333333333,0.333333333333333,0.333333333333333,
0.333333333333333,0.333333333333333,0.333333333333333,0.333333333333333,
0.333333333333333,0.333333333333333,0.333333333333333,0.333333333333333,
0.333333333333333,0.333333333333333,0.333333333333333,0.333333333333333,
0.333333333333333,0.333333333333333,0.333333333333333,0.333333333333333,
0.333333333333333,0.333333333333333,0.333333333333333,0.333333333333333,
0.333333333333333,0.333333333333333,0.333333333333333,0.333333333333333,
0.333333333333333,0.333333333333333,0.333333333333333,0.333333333333333,
0.333333333333333,0.333333333333333,0.333333333333333,0.333333333333333,
0.333333333333333,0.333333333333333,0.333333333333333,0.333333333333333,
0.333333333333333,0.333333333333333,0.333333333333333,0.333333333333333,
0.333333333333333),(1.,1.,1.,1.,1.,1.,1.,1.,1.,1.,1.,1.,1.,1.,1.,1.,1.,
1.,1.,1.,1.,1.,1.,1.,1.,1.,1.,1.,1.,1.,1.,1.,1.,1.,1.,1.,1.,1.,1.,1.,1.,
1.,1.,1.,1.,1.,1.,1.,1.,1.,1.,1.,1.,1.,1.,1.,1.,1.,1.,1.,1.,1.,1.,1.,1.,
1.,1.,1.,1.,1.,1.,1.,1.,1.,1.,1.,1.,1.,1.,1.,1.,1.,1.,1.,1.,1.,1.,1.,1.,
1.,1.,1.,1.,1.,1.,1.,1.,1.,1.,1.,1.,1.,1.,1.,1.,1.,1.,1.,1.,1.,1.,1.,1.,
1.,1.,1.,1.,1.,1.,1.,1.,1.,1.,1.,1.,1.,1.,1.,1.,1.,1.,1.,1.,1.,1.,1.,1.,
1.,1.,1.,1.,1.,1.,1.,1.,1.,1.,1.,1.,1.,1.,1.,1.,1.,1.,1.,1.,1.,1.,1.,1.,
1.,1.,1.,1.,1.,1.,1.),(0.333333333333333,0.333333333333333,0.333333333333333,
0.333333333333333,0.333333333333333,0.333333333333333,0.333333333333333,
0.333333333333333,0.333333333333333,0.333333333333333,0.333333333333333,
0.333333333333333,0.333333333333333,0.333333333333333,0.333333333333333,
0.333333333333333,0.333333333333333,0.333333333333333,0.333333333333333,
0.333333333333333,0.333333333333333,0.333333333333333,0.333333333333333,
0.333333333333333,0.333333333333333,0.333333333333333,0.333333333333333,
0.333333333333333,0.333333333333333,0.333333333333333,0.333333333333333,
0.333333333333333,0.333333333333333,0.333333333333333,0.333333333333333,
0.333333333333333,0.333333333333333,0.333333333333333,0.333333333333333,
0.333333333333333,0.333333333333333,0.333333333333333,0.333333333333333,
0.333333333333333,0.333333333333333,0.333333333333333,0.333333333333333,
0.333333333333333,0.333333333333333,0.333333333333333,0.333333333333333,
0.333333333333333,0.333333333333333,0.333333333333333,0.333333333333333,
0.333333333333333,0.333333333333333,0.333333333333333,0.333333333333333,
0.333333333333333,0.333333333333333,0.333333333333333,0.333333333333333,
0.333333333333333,0.333333333333333,0.333333333333333,0.333333333333333,
0.333333333333333,0.333333333333333,0.333333333333333,0.333333333333333,
0.333333333333333,0.333333333333333,0.333333333333333,0.333333333333333,
0.333333333333333,0.333333333333333,0.333333333333333,0.333333333333333,
0.333333333333333,0.333333333333333,0.333333333333333,0.333333333333333,
0.333333333333333,0.333333333333333,0.333333333333333,0.333333333333333,
0.333333333333333,0.333333333333333,0.333333333333333,0.333333333333333,
0.333333333333333,0.333333333333333,0.333333333333333,0.333333333333333,
0.333333333333333,0.333333333333333,0.333333333333333,0.333333333333333,
0.333333333333333,0.333333333333333,0.333333333333333,0.333333333333333,
0.333333333333333,0.333333333333333,0.333333333333333,0.333333333333333,
0.333333333333333,0.333333333333333,0.333333333333333,0.333333333333333,
0.333333333333333,0.333333333333333,0.333333333333333,0.333333333333333,
0.333333333333333,0.333333333333333,0.333333333333333,0.333333333333333,
0.333333333333333,0.333333333333333,0.333333333333333,0.333333333333333,
0.333333333333333,0.333333333333333,0.333333333333333,0.333333333333333,
0.333333333333333,0.333333333333333,0.333333333333333,0.333333333333333,
0.333333333333333,0.333333333333333,0.333333333333333,0.333333333333333,
0.333333333333333,0.333333333333333,0.333333333333333,0.333333333333333,
0.333333333333333,0.333333333333333,0.333333333333333,0.333333333333333,
0.333333333333333,0.333333333333333,0.333333333333333,0.333333333333333,
0.333333333333333,0.333333333333333,0.333333333333333,0.333333333333333,
0.333333333333333,0.333333333333333,0.333333333333333,0.333333333333333,
0.333333333333333,0.333333333333333,0.333333333333333,0.333333333333333,
0.333333333333333,0.333333333333333,0.333333333333333,0.333333333333333,
0.333333333333333,0.333333333333333,0.333333333333333,0.333333333333333,
0.333333333333333),(0.333333333333333,0.333333333333333,0.333333333333333,
0.333333333333333,0.333333333333333,0.333333333333333,0.333333333333333,
0.333333333333333,0.333333333333333,0.333333333333333,0.333333333333333,
0.333333333333333,0.333333333333333,0.333333333333333,0.333333333333333,
0.333333333333333,0.333333333333333,0.333333333333333,0.333333333333333,
0.333333333333333,0.333333333333333,0.333333333333333,0.333333333333333,
0.333333333333333,0.333333333333333,0.333333333333333,0.333333333333333,
0.333333333333333,0.333333333333333,0.333333333333333,0.333333333333333,
0.333333333333333,0.333333333333333,0.333333333333333,0.333333333333333,
0.333333333333333,0.333333333333333,0.333333333333333,0.333333333333333,
0.333333333333333,0.333333333333333,0.333333333333333,0.333333333333333,
0.333333333333333,0.333333333333333,0.333333333333333,0.333333333333333,
0.333333333333333,0.333333333333333,0.333333333333333,0.333333333333333,
0.333333333333333,0.333333333333333,0.333333333333333,0.333333333333333,
0.333333333333333,0.333333333333333,0.333333333333333,0.333333333333333,
0.333333333333333,0.333333333333333,0.333333333333333,0.333333333333333,
0.333333333333333,0.333333333333333,0.333333333333333,0.333333333333333,
0.333333333333333,0.333333333333333,0.333333333333333,0.333333333333333,
0.333333333333333,0.333333333333333,0.333333333333333,0.333333333333333,
0.333333333333333,0.333333333333333,0.333333333333333,0.333333333333333,
0.333333333333333,0.333333333333333,0.333333333333333,0.333333333333333,
0.333333333333333,0.333333333333333,0.333333333333333,0.333333333333333,
0.333333333333333,0.333333333333333,0.333333333333333,0.333333333333333,
0.333333333333333,0.333333333333333,0.333333333333333,0.333333333333333,
0.333333333333333,0.333333333333333,0.333333333333333,0.333333333333333,
0.333333333333333,0.333333333333333,0.333333333333333,0.333333333333333,
0.333333333333333,0.333333333333333,0.333333333333333,0.333333333333333,
0.333333333333333,0.333333333333333,0.333333333333333,0.333333333333333,
0.333333333333333,0.333333333333333,0.333333333333333,0.333333333333333,
0.333333333333333,0.333333333333333,0.333333333333333,0.333333333333333,
0.333333333333333,0.333333333333333,0.333333333333333,0.333333333333333,
0.333333333333333,0.333333333333333,0.333333333333333,0.333333333333333,
0.333333333333333,0.333333333333333,0.333333333333333,0.333333333333333,
0.333333333333333,0.333333333333333,0.333333333333333,0.333333333333333,
0.333333333333333,0.333333333333333,0.333333333333333,0.333333333333333,
0.333333333333333,0.333333333333333,0.333333333333333,0.333333333333333,
0.333333333333333,0.333333333333333,0.333333333333333,0.333333333333333,
0.333333333333333,0.333333333333333,0.333333333333333,0.333333333333333,
0.333333333333333,0.333333333333333,0.333333333333333,0.333333333333333,
0.333333333333333,0.333333333333333,0.333333333333333,0.333333333333333,
0.333333333333333,0.333333333333333,0.333333333333333,0.333333333333333,
0.333333333333333,0.333333333333333,0.333333333333333,0.333333333333333,
0.333333333333333),(1.,1.,1.,1.,1.,1.,1.,1.,1.,1.,1.,1.,1.,1.,1.,1.,1.,
1.,1.,1.,1.,1.,1.,1.,1.,1.,1.,1.,1.,1.,1.,1.,1.,1.,1.,1.,1.,1.,1.,1.,1.,
1.,1.,1.,1.,1.,1.,1.,1.,1.,1.,1.,1.,1.,1.,1.,1.,1.,1.,1.,1.,1.,1.,1.,1.,
1.,1.,1.,1.,1.,1.,1.,1.,1.,1.,1.,1.,1.,1.,1.,1.,1.,1.,1.,1.,1.,1.,1.,1.,
1.,1.,1.,1.,1.,1.,1.,1.,1.,1.,1.,1.,1.,1.,1.,1.,1.,1.,1.,1.,1.,1.,1.,1.,
1.,1.,1.,1.,1.,1.,1.,1.,1.,1.,1.,1.,1.,1.,1.,1.,1.,1.,1.,1.,1.,1.,1.,1.,
1.,1.,1.,1.,1.,1.,1.,1.,1.,1.,1.,1.,1.,1.,1.,1.,1.,1.,1.,1.,1.,1.,1.,1.,
1.,1.,1.,1.,1.,1.,1.)))
REPRESENTATION_ITEM('')
SURFACE()
);
#531=(
BOUNDED_SURFACE()
B_SPLINE_SURFACE(3,3,((#15532,#15533,#15534,#15535,#15536,#15537,#15538,
#15539,#15540,#15541,#15542,#15543,#15544,#15545,#15546,#15547,#15548,#15549,
#15550,#15551),(#15552,#15553,#15554,#15555,#15556,#15557,#15558,#15559,
#15560,#15561,#15562,#15563,#15564,#15565,#15566,#15567,#15568,#15569,#15570,
#15571),(#15572,#15573,#15574,#15575,#15576,#15577,#15578,#15579,#15580,
#15581,#15582,#15583,#15584,#15585,#15586,#15587,#15588,#15589,#15590,#15591),
(#15592,#15593,#15594,#15595,#15596,#15597,#15598,#15599,#15600,#15601,
#15602,#15603,#15604,#15605,#15606,#15607,#15608,#15609,#15610,#15611),
(#15612,#15613,#15614,#15615,#15616,#15617,#15618,#15619,#15620,#15621,
#15622,#15623,#15624,#15625,#15626,#15627,#15628,#15629,#15630,#15631),
(#15632,#15633,#15634,#15635,#15636,#15637,#15638,#15639,#15640,#15641,
#15642,#15643,#15644,#15645,#15646,#15647,#15648,#15649,#15650,#15651),
(#15652,#15653,#15654,#15655,#15656,#15657,#15658,#15659,#15660,#15661,
#15662,#15663,#15664,#15665,#15666,#15667,#15668,#15669,#15670,#15671)),
 .UNSPECIFIED.,.T.,.F.,.F.)
B_SPLINE_SURFACE_WITH_KNOTS((4,3,4),(4,2,2,2,2,2,2,2,2,4),(0.,0.5,1.),(0.0618954463697512,
0.0653601604005303,0.0688248744313094,0.0757543024928677,0.0792190165236468,
0.0809513735390363,0.0826837305544259,0.086148444585205,0.0878808016005946,
0.0896131586159842),.UNSPECIFIED.)
GEOMETRIC_REPRESENTATION_ITEM()
RATIONAL_B_SPLINE_SURFACE(((1.,1.,1.,1.,1.,1.,1.,1.,1.,1.,1.,1.,1.,1.,1.,
1.,1.,1.,1.,1.),(0.333333333333333,0.333333333333333,0.333333333333333,
0.333333333333333,0.333333333333333,0.333333333333333,0.333333333333333,
0.333333333333333,0.333333333333333,0.333333333333333,0.333333333333333,
0.333333333333333,0.333333333333333,0.333333333333333,0.333333333333333,
0.333333333333333,0.333333333333333,0.333333333333333,0.333333333333333,
0.333333333333333),(0.333333333333333,0.333333333333333,0.333333333333333,
0.333333333333333,0.333333333333333,0.333333333333333,0.333333333333333,
0.333333333333333,0.333333333333333,0.333333333333333,0.333333333333333,
0.333333333333333,0.333333333333333,0.333333333333333,0.333333333333333,
0.333333333333333,0.333333333333333,0.333333333333333,0.333333333333333,
0.333333333333333),(1.,1.,1.,1.,1.,1.,1.,1.,1.,1.,1.,1.,1.,1.,1.,1.,1.,
1.,1.,1.),(0.333333333333333,0.333333333333333,0.333333333333333,0.333333333333333,
0.333333333333333,0.333333333333333,0.333333333333333,0.333333333333333,
0.333333333333333,0.333333333333333,0.333333333333333,0.333333333333333,
0.333333333333333,0.333333333333333,0.333333333333333,0.333333333333333,
0.333333333333333,0.333333333333333,0.333333333333333,0.333333333333333),
(0.333333333333333,0.333333333333333,0.333333333333333,0.333333333333333,
0.333333333333333,0.333333333333333,0.333333333333333,0.333333333333333,
0.333333333333333,0.333333333333333,0.333333333333333,0.333333333333333,
0.333333333333333,0.333333333333333,0.333333333333333,0.333333333333333,
0.333333333333333,0.333333333333333,0.333333333333333,0.333333333333333),
(1.,1.,1.,1.,1.,1.,1.,1.,1.,1.,1.,1.,1.,1.,1.,1.,1.,1.,1.,1.)))
REPRESENTATION_ITEM('')
SURFACE()
);
#606=TOROIDAL_SURFACE('',#9082,2.00000000000001,0.4);
#607=TOROIDAL_SURFACE('',#9088,2.,0.4);
#608=TOROIDAL_SURFACE('',#9093,1.79999999999999,0.4);
#609=TOROIDAL_SURFACE('',#9096,1.8,0.4);
#675=SHAPE_REPRESENTATION_RELATIONSHIP('SRR','None',#47762,#687);
#687=ADVANCED_BREP_SHAPE_REPRESENTATION('',(#711),#47706);
#699=STYLED_ITEM('',(#47830),#711);
#711=MANIFOLD_SOLID_BREP('Body1',#8926);
#761=PLANE('',#9110);
#762=PLANE('',#9111);
#884=LINE('',#12260,#1371);
#885=LINE('',#14184,#1372);
#1371=VECTOR('',#10017,0.400000000000003);
#1372=VECTOR('',#10032,0.400000000000011);
#1858=CYLINDRICAL_SURFACE('',#9099,0.400000000000003);
#1859=CYLINDRICAL_SURFACE('',#9106,0.400000000000011);
#2068=FACE_OUTER_BOUND('',#2582,.T.);
#2069=FACE_OUTER_BOUND('',#2583,.T.);
#2070=FACE_OUTER_BOUND('',#2584,.T.);
#2071=FACE_OUTER_BOUND('',#2585,.T.);
#2072=FACE_OUTER_BOUND('',#2586,.T.);
#2073=FACE_OUTER_BOUND('',#2587,.T.);
#2074=FACE_OUTER_BOUND('',#2588,.T.);
#2075=FACE_OUTER_BOUND('',#2589,.T.);
#2076=FACE_OUTER_BOUND('',#2590,.T.);
#2077=FACE_OUTER_BOUND('',#2591,.T.);
#2078=FACE_OUTER_BOUND('',#2592,.T.);
#2079=FACE_OUTER_BOUND('',#2593,.T.);
#2080=FACE_OUTER_BOUND('',#2594,.T.);
#2081=FACE_OUTER_BOUND('',#2595,.T.);
#2582=EDGE_LOOP('',(#5737,#5738,#5739,#5740,#5741,#5742));
#2583=EDGE_LOOP('',(#5743,#5744,#5745,#5746,#5747));
#2584=EDGE_LOOP('',(#5748,#5749,#5750,#5751,#5752));
#2585=EDGE_LOOP('',(#5753,#5754,#5755,#5756,#5757));
#2586=EDGE_LOOP('',(#5758,#5759,#5760,#5761,#5762,#5763,#5764));
#2587=EDGE_LOOP('',(#5765,#5766,#5767,#5768));
#2588=EDGE_LOOP('',(#5769,#5770,#5771,#5772));
#2589=EDGE_LOOP('',(#5773,#5774,#5775,#5776));
#2590=EDGE_LOOP('',(#5777,#5778,#5779,#5780,#5781));
#2591=EDGE_LOOP('',(#5782,#5783,#5784,#5785,#5786));
#2592=EDGE_LOOP('',(#5787,#5788,#5789,#5790));
#2593=EDGE_LOOP('',(#5791,#5792,#5793,#5794));
#2594=EDGE_LOOP('',(#5795));
#2595=EDGE_LOOP('',(#5796));
#3128=CIRCLE('',#9083,0.400000000000007);
#3129=CIRCLE('',#9084,0.400000000000007);
#3130=CIRCLE('',#9085,1.6);
#3131=CIRCLE('',#9086,0.400000000000014);
#3132=CIRCLE('',#9087,0.400000000000014);
#3133=CIRCLE('',#9089,0.400000000000011);
#3134=CIRCLE('',#9090,1.6);
#3135=CIRCLE('',#9091,0.399999999999994);
#3136=CIRCLE('',#9092,0.399999999999994);
#3137=CIRCLE('',#9094,1.39999999999999);
#3138=CIRCLE('',#9095,0.399999999999997);
#3139=CIRCLE('',#9097,0.400000000000009);
#3140=CIRCLE('',#9098,1.4);
#3141=CIRCLE('',#9100,0.400000000000014);
#3142=CIRCLE('',#9101,0.400000000000014);
#3143=CIRCLE('',#9102,0.400000000000014);
#3144=CIRCLE('',#9103,0.400000000000013);
#3145=CIRCLE('',#9104,0.399999999999995);
#3146=CIRCLE('',#9105,0.400000000000011);
#3147=CIRCLE('',#9107,0.400000000000011);
#3148=CIRCLE('',#9108,0.400000000000013);
#3149=CIRCLE('',#9109,0.399999999999995);
#3536=VERTEX_POINT('',#12233);
#3537=VERTEX_POINT('',#12234);
#3538=VERTEX_POINT('',#12237);
#3539=VERTEX_POINT('',#12239);
#3540=VERTEX_POINT('',#12243);
#3541=VERTEX_POINT('',#12245);
#3542=VERTEX_POINT('',#12247);
#3543=VERTEX_POINT('',#12251);
#3544=VERTEX_POINT('',#12255);
#3545=VERTEX_POINT('',#12259);
#3546=VERTEX_POINT('',#12261);
#3547=VERTEX_POINT('',#12263);
#3548=VERTEX_POINT('',#12434);
#3549=VERTEX_POINT('',#12435);
#3550=VERTEX_POINT('',#13661);
#3551=VERTEX_POINT('',#13662);
#3552=VERTEX_POINT('',#14140);
#3553=VERTEX_POINT('',#14141);
#4394=EDGE_CURVE('',#3536,#3537,#3128,.T.);
#4395=EDGE_CURVE('',#3537,#3536,#3129,.T.);
#4396=EDGE_CURVE('',#3536,#3538,#3130,.T.);
#4397=EDGE_CURVE('',#3539,#3538,#3131,.T.);
#4398=EDGE_CURVE('',#3538,#3539,#3132,.T.);
#4399=EDGE_CURVE('',#3540,#3540,#3133,.T.);
#4400=EDGE_CURVE('',#3540,#3541,#3134,.T.);
#4401=EDGE_CURVE('',#3542,#3541,#3135,.T.);
#4402=EDGE_CURVE('',#3541,#3542,#3136,.T.);
#4403=EDGE_CURVE('',#3542,#3543,#3137,.T.);
#4404=EDGE_CURVE('',#3543,#3543,#3138,.T.);
#4405=EDGE_CURVE('',#3544,#3544,#3139,.T.);
#4406=EDGE_CURVE('',#3544,#3537,#3140,.T.);
#4407=EDGE_CURVE('',#3539,#3545,#884,.T.);
#4408=EDGE_CURVE('',#3546,#3545,#3141,.T.);
#4409=EDGE_CURVE('',#3547,#3546,#3142,.T.);
#4410=EDGE_CURVE('',#3545,#3547,#3143,.T.);
#4411=EDGE_CURVE('',#3548,#3549,#3144,.T.);
#4412=EDGE_CURVE('',#3548,#3547,#148,.T.);
#4413=EDGE_CURVE('',#3549,#3546,#149,.T.);
#4414=EDGE_CURVE('',#3550,#3551,#3145,.T.);
#4415=EDGE_CURVE('',#3550,#3548,#150,.T.);
#4416=EDGE_CURVE('',#3551,#3549,#151,.T.);
#4417=EDGE_CURVE('',#3552,#3553,#3146,.T.);
#4418=EDGE_CURVE('',#3552,#3550,#152,.T.);
#4419=EDGE_CURVE('',#3553,#3551,#153,.T.);
#4420=EDGE_CURVE('',#3553,#3540,#885,.T.);
#4421=EDGE_CURVE('',#3553,#3552,#3147,.T.);
#4422=EDGE_CURVE('',#3549,#3548,#3148,.T.);
#4423=EDGE_CURVE('',#3551,#3550,#3149,.T.);
#5737=ORIENTED_EDGE('',*,*,#4394,.T.);
#5738=ORIENTED_EDGE('',*,*,#4395,.T.);
#5739=ORIENTED_EDGE('',*,*,#4396,.T.);
#5740=ORIENTED_EDGE('',*,*,#4397,.F.);
#5741=ORIENTED_EDGE('',*,*,#4398,.F.);
#5742=ORIENTED_EDGE('',*,*,#4396,.F.);
#5743=ORIENTED_EDGE('',*,*,#4399,.T.);
#5744=ORIENTED_EDGE('',*,*,#4400,.T.);
#5745=ORIENTED_EDGE('',*,*,#4401,.F.);
#5746=ORIENTED_EDGE('',*,*,#4402,.F.);
#5747=ORIENTED_EDGE('',*,*,#4400,.F.);
#5748=ORIENTED_EDGE('',*,*,#4402,.T.);
#5749=ORIENTED_EDGE('',*,*,#4403,.T.);
#5750=ORIENTED_EDGE('',*,*,#4404,.F.);
#5751=ORIENTED_EDGE('',*,*,#4403,.F.);
#5752=ORIENTED_EDGE('',*,*,#4401,.T.);
#5753=ORIENTED_EDGE('',*,*,#4405,.T.);
#5754=ORIENTED_EDGE('',*,*,#4406,.T.);
#5755=ORIENTED_EDGE('',*,*,#4394,.F.);
#5756=ORIENTED_EDGE('',*,*,#4395,.F.);
#5757=ORIENTED_EDGE('',*,*,#4406,.F.);
#5758=ORIENTED_EDGE('',*,*,#4397,.T.);
#5759=ORIENTED_EDGE('',*,*,#4398,.T.);
#5760=ORIENTED_EDGE('',*,*,#4407,.T.);
#5761=ORIENTED_EDGE('',*,*,#4408,.F.);
#5762=ORIENTED_EDGE('',*,*,#4409,.F.);
#5763=ORIENTED_EDGE('',*,*,#4410,.F.);
#5764=ORIENTED_EDGE('',*,*,#4407,.F.);
#5765=ORIENTED_EDGE('',*,*,#4411,.F.);
#5766=ORIENTED_EDGE('',*,*,#4412,.T.);
#5767=ORIENTED_EDGE('',*,*,#4409,.T.);
#5768=ORIENTED_EDGE('',*,*,#4413,.F.);
#5769=ORIENTED_EDGE('',*,*,#4414,.F.);
#5770=ORIENTED_EDGE('',*,*,#4415,.T.);
#5771=ORIENTED_EDGE('',*,*,#4411,.T.);
#5772=ORIENTED_EDGE('',*,*,#4416,.F.);
#5773=ORIENTED_EDGE('',*,*,#4417,.F.);
#5774=ORIENTED_EDGE('',*,*,#4418,.T.);
#5775=ORIENTED_EDGE('',*,*,#4414,.T.);
#5776=ORIENTED_EDGE('',*,*,#4419,.F.);
#5777=ORIENTED_EDGE('',*,*,#4417,.T.);
#5778=ORIENTED_EDGE('',*,*,#4420,.T.);
#5779=ORIENTED_EDGE('',*,*,#4399,.F.);
#5780=ORIENTED_EDGE('',*,*,#4420,.F.);
#5781=ORIENTED_EDGE('',*,*,#4421,.T.);
#5782=ORIENTED_EDGE('',*,*,#4412,.F.);
#5783=ORIENTED_EDGE('',*,*,#4422,.F.);
#5784=ORIENTED_EDGE('',*,*,#4413,.T.);
#5785=ORIENTED_EDGE('',*,*,#4408,.T.);
#5786=ORIENTED_EDGE('',*,*,#4410,.T.);
#5787=ORIENTED_EDGE('',*,*,#4415,.F.);
#5788=ORIENTED_EDGE('',*,*,#4423,.F.);
#5789=ORIENTED_EDGE('',*,*,#4416,.T.);
#5790=ORIENTED_EDGE('',*,*,#4422,.T.);
#5791=ORIENTED_EDGE('',*,*,#4418,.F.);
#5792=ORIENTED_EDGE('',*,*,#4421,.F.);
#5793=ORIENTED_EDGE('',*,*,#4419,.T.);
#5794=ORIENTED_EDGE('',*,*,#4423,.T.);
#5795=ORIENTED_EDGE('',*,*,#4405,.F.);
#5796=ORIENTED_EDGE('',*,*,#4404,.T.);
#8418=ADVANCED_FACE('',(#2068),#606,.T.);
#8419=ADVANCED_FACE('',(#2069),#607,.T.);
#8420=ADVANCED_FACE('',(#2070),#608,.T.);
#8421=ADVANCED_FACE('',(#2071),#609,.T.);
#8422=ADVANCED_FACE('',(#2072),#1858,.T.);
#8423=ADVANCED_FACE('',(#2073),#526,.F.);
#8424=ADVANCED_FACE('',(#2074),#527,.F.);
#8425=ADVANCED_FACE('',(#2075),#528,.F.);
#8426=ADVANCED_FACE('',(#2076),#1859,.T.);
#8427=ADVANCED_FACE('',(#2077),#529,.F.);
#8428=ADVANCED_FACE('',(#2078),#530,.F.);
#8429=ADVANCED_FACE('',(#2079),#531,.F.);
#8430=ADVANCED_FACE('',(#2080),#761,.F.);
#8431=ADVANCED_FACE('',(#2081),#762,.T.);
#8926=CLOSED_SHELL('',(#8418,#8419,#8420,#8421,#8422,#8423,#8424,#8425,
#8426,#8427,#8428,#8429,#8430,#8431));
#9081=AXIS2_PLACEMENT_3D('',#12231,#9979,#9980);
#9082=AXIS2_PLACEMENT_3D('',#12232,#9981,#9982);
#9083=AXIS2_PLACEMENT_3D('',#12235,#9983,#9984);
#9084=AXIS2_PLACEMENT_3D('',#12236,#9985,#9986);
#9085=AXIS2_PLACEMENT_3D('',#12238,#9987,#9988);
#9086=AXIS2_PLACEMENT_3D('',#12240,#9989,#9990);
#9087=AXIS2_PLACEMENT_3D('',#12241,#9991,#9992);
#9088=AXIS2_PLACEMENT_3D('',#12242,#9993,#9994);
#9089=AXIS2_PLACEMENT_3D('',#12244,#9995,#9996);
#9090=AXIS2_PLACEMENT_3D('',#12246,#9997,#9998);
#9091=AXIS2_PLACEMENT_3D('',#12248,#9999,#10000);
#9092=AXIS2_PLACEMENT_3D('',#12249,#10001,#10002);
#9093=AXIS2_PLACEMENT_3D('',#12250,#10003,#10004);
#9094=AXIS2_PLACEMENT_3D('',#12252,#10005,#10006);
#9095=AXIS2_PLACEMENT_3D('',#12253,#10007,#10008);
#9096=AXIS2_PLACEMENT_3D('',#12254,#10009,#10010);
#9097=AXIS2_PLACEMENT_3D('',#12256,#10011,#10012);
#9098=AXIS2_PLACEMENT_3D('',#12257,#10013,#10014);
#9099=AXIS2_PLACEMENT_3D('',#12258,#10015,#10016);
#9100=AXIS2_PLACEMENT_3D('',#12262,#10018,#10019);
#9101=AXIS2_PLACEMENT_3D('',#12264,#10020,#10021);
#9102=AXIS2_PLACEMENT_3D('',#12265,#10022,#10023);
#9103=AXIS2_PLACEMENT_3D('',#12436,#10024,#10025);
#9104=AXIS2_PLACEMENT_3D('',#13663,#10026,#10027);
#9105=AXIS2_PLACEMENT_3D('',#14142,#10028,#10029);
#9106=AXIS2_PLACEMENT_3D('',#14183,#10030,#10031);
#9107=AXIS2_PLACEMENT_3D('',#14185,#10033,#10034);
#9108=AXIS2_PLACEMENT_3D('',#14354,#10035,#10036);
#9109=AXIS2_PLACEMENT_3D('',#15531,#10037,#10038);
#9110=AXIS2_PLACEMENT_3D('',#15672,#10039,#10040);
#9111=AXIS2_PLACEMENT_3D('',#15673,#10041,#10042);
#9979=DIRECTION('axis',(0.,0.,1.));
#9980=DIRECTION('refdir',(1.,0.,0.));
#9981=DIRECTION('center_axis',(0.981909603155918,0.18935028711409,1.69243964532307E-17));
#9982=DIRECTION('ref_axis',(0.,9.25185853854295E-17,-1.));
#9983=DIRECTION('center_axis',(0.099658045849521,-0.516794527976799,-0.850289180073869));
#9984=DIRECTION('ref_axis',(-0.177993700909268,-0.850018762193619,0.495768440257597));
#9985=DIRECTION('center_axis',(0.099658045849521,-0.516794527976799,-0.850289180073869));
#9986=DIRECTION('ref_axis',(-0.177993700909268,-0.850018762193619,0.495768440257597));
#9987=DIRECTION('center_axis',(-0.981909603155918,-0.18935028711409,-1.69243964532307E-17));
#9988=DIRECTION('ref_axis',(4.91815976796491E-19,8.68310150104084E-17,-1.));
#9989=DIRECTION('center_axis',(0.18935028711409,-0.981909603155918,4.32306217395459E-16));
#9990=DIRECTION('ref_axis',(-0.329651622039256,-0.063569629098379,0.941960036489437));
#9991=DIRECTION('center_axis',(0.18935028711409,-0.981909603155918,4.32306217395459E-16));
#9992=DIRECTION('ref_axis',(-0.329651622039256,-0.063569629098379,0.941960036489437));
#9993=DIRECTION('center_axis',(-0.981909603155918,-0.18935028711409,-1.69243964532307E-17));
#9994=DIRECTION('ref_axis',(0.,0.,1.));
#9995=DIRECTION('center_axis',(0.18935028711409,-0.981909603155918,-6.2240565599844E-16));
#9996=DIRECTION('ref_axis',(-1.17852689664738E-16,6.11146090683426E-16,
-1.));
#9997=DIRECTION('center_axis',(0.981909603155918,0.18935028711409,1.69243964532307E-17));
#9998=DIRECTION('ref_axis',(-1.66182274050451E-17,-3.20463932765191E-18,
1.));
#9999=DIRECTION('center_axis',(0.0996580458495207,-0.516794527976797,-0.85028918007387));
#10000=DIRECTION('ref_axis',(-0.161002500376988,0.834907111374105,-0.526315789473682));
#10001=DIRECTION('center_axis',(0.0996580458495207,-0.516794527976797,-0.85028918007387));
#10002=DIRECTION('ref_axis',(-0.161002500376988,0.834907111374105,-0.526315789473682));
#10003=DIRECTION('center_axis',(0.981909603155918,0.18935028711409,1.69243964532307E-17));
#10004=DIRECTION('ref_axis',(0.188087212577509,-0.975359705419448,-0.115311081466222));
#10005=DIRECTION('center_axis',(-0.981909603155918,-0.18935028711409,-1.69243964532307E-17));
#10006=DIRECTION('ref_axis',(0.188087212577511,-0.975359705419448,-0.115311081466224));
#10007=DIRECTION('center_axis',(-0.133890872037992,0.694314938903739,-0.70710678118655));
#10008=DIRECTION('ref_axis',(-0.133890872037987,0.694314938903745,0.707106781186545));
#10009=DIRECTION('center_axis',(-0.981909603155918,-0.18935028711409,-1.69243964532307E-17));
#10010=DIRECTION('ref_axis',(-0.188087212577509,0.975359705419448,0.115311081466222));
#10011=DIRECTION('center_axis',(-0.133890872037992,0.694314938903738,-0.707106781186551));
#10012=DIRECTION('ref_axis',(-0.203531771328762,-0.717586554283311,-0.666066329408401));
#10013=DIRECTION('center_axis',(0.981909603155918,0.18935028711409,1.69243964532307E-17));
#10014=DIRECTION('ref_axis',(-0.188087212577511,0.975359705419448,0.115311081466223));
#10015=DIRECTION('center_axis',(-0.18935028711409,0.981909603155918,6.72941436858614E-17));
#10016=DIRECTION('ref_axis',(0.981909603155918,0.18935028711409,8.26841968029962E-32));
#10017=DIRECTION('',(0.18935028711409,-0.981909603155918,-6.72941436858614E-17));
#10018=DIRECTION('center_axis',(0.18935028711409,-0.981909603155918,4.32306217395459E-16));
#10019=DIRECTION('ref_axis',(-0.329651622039256,-0.063569629098379,0.941960036489437));
#10020=DIRECTION('center_axis',(0.18935028711409,-0.981909603155918,4.32306217395459E-16));
#10021=DIRECTION('ref_axis',(-0.329651622039256,-0.063569629098379,0.941960036489437));
#10022=DIRECTION('center_axis',(0.18935028711409,-0.981909603155918,4.32306217395459E-16));
#10023=DIRECTION('ref_axis',(-0.329651622039256,-0.063569629098379,0.941960036489437));
#10024=DIRECTION('center_axis',(-0.650733917652094,-0.302831987743225,-0.696303206668362));
#10025=DIRECTION('ref_axis',(-0.734158582489553,0.484984699073061,0.475185245374835));
#10026=DIRECTION('center_axis',(-0.650733917651975,-0.302831987743205,-0.696303206668483));
#10027=DIRECTION('ref_axis',(-0.734238772574636,0.484644912666334,0.475407965304257));
#10028=DIRECTION('center_axis',(0.18935028711409,-0.981909603155918,1.5475046123917E-16));
#10029=DIRECTION('ref_axis',(2.93020442666747E-17,-1.51950963983549E-16,
-1.));
#10030=DIRECTION('center_axis',(-0.18935028711409,0.981909603155918,-7.59938514614303E-16));
#10031=DIRECTION('ref_axis',(-1.43894575931273E-16,7.46190925307827E-16,
1.));
#10032=DIRECTION('',(0.18935028711409,-0.981909603155918,7.59938514614303E-16));
#10033=DIRECTION('center_axis',(0.18935028711409,-0.981909603155918,1.5475046123917E-16));
#10034=DIRECTION('ref_axis',(2.93020442666747E-17,-1.51950963983549E-16,
-1.));
#10035=DIRECTION('center_axis',(-0.650733917652094,-0.302831987743225,-0.696303206668362));
#10036=DIRECTION('ref_axis',(-0.734158582489553,0.484984699073061,0.475185245374835));
#10037=DIRECTION('center_axis',(-0.650733917651975,-0.302831987743205,-0.696303206668483));
#10038=DIRECTION('ref_axis',(-0.734238772574636,0.484644912666334,0.475407965304257));
#10039=DIRECTION('center_axis',(-0.133890872037992,0.694314938903738,-0.707106781186551));
#10040=DIRECTION('ref_axis',(-0.203531771328761,-0.717586554283311,-0.666066329408402));
#10041=DIRECTION('center_axis',(-0.133890872037992,0.694314938903739,-0.70710678118655));
#10042=DIRECTION('ref_axis',(-0.133890872037993,0.694314938903744,0.707106781186545));
#12231=CARTESIAN_POINT('',(0.,0.,0.));
#12232=CARTESIAN_POINT('Origin',(-54.1881478197433,0.967499828069326,177.985485069079));
#12233=CARTESIAN_POINT('',(-54.4457518203465,2.3033512062679,177.143379805922));
#12234=CARTESIAN_POINT('',(-54.5745538206481,2.97127689536718,176.722327174343));
#12235=CARTESIAN_POINT('Origin',(-54.5101528204973,2.63731405081754,176.932853490132));
#12236=CARTESIAN_POINT('Origin',(-54.5101528204973,2.63731405081754,176.932853490132));
#12237=CARTESIAN_POINT('',(-54.1881478197433,0.967499828069329,176.385485069079));
#12238=CARTESIAN_POINT('Origin',(-54.1881478197433,0.967499828069326,177.985485069079));
#12239=CARTESIAN_POINT('',(-54.5809116610057,0.891759713223694,175.985485069079));
#12240=CARTESIAN_POINT('Origin',(-54.1881478197433,0.967499828069329,175.985485069079));
#12241=CARTESIAN_POINT('Origin',(-54.1881478197433,0.967499828069329,175.985485069079));
#12242=CARTESIAN_POINT('Origin',(-47.8413342697331,-31.9450310646891,173.985485069079));
#12243=CARTESIAN_POINT('',(-47.8413342697331,-31.9450310646891,175.585485069079));
#12244=CARTESIAN_POINT('Origin',(-47.8413342697331,-31.9450310646891,175.985485069079));
#12245=CARTESIAN_POINT('',(-47.5837302691299,-33.2808824428876,174.827590332237));
#12246=CARTESIAN_POINT('Origin',(-47.8413342697331,-31.9450310646891,173.985485069079));
#12247=CARTESIAN_POINT('',(-47.4549282688283,-33.9488081319869,175.248642963816));
#12248=CARTESIAN_POINT('Origin',(-47.5193292689791,-33.6148452874373,175.038116648027));
#12249=CARTESIAN_POINT('Origin',(-47.5193292689791,-33.6148452874373,175.038116648027));
#12250=CARTESIAN_POINT('Origin',(-47.2295247683005,-35.1176780879106,175.985485069079));
#12251=CARTESIAN_POINT('',(-47.4169719891537,-34.1456371734454,176.975434562741));
#12252=CARTESIAN_POINT('Origin',(-47.2295247683005,-35.1176780879106,175.985485069079));
#12253=CARTESIAN_POINT('Origin',(-47.4705283379689,-33.8679111978839,177.258277275215));
#12254=CARTESIAN_POINT('Origin',(-54.7999573211759,4.14014685129092,175.985485069079));
#12255=CARTESIAN_POINT('',(-54.6125101003227,3.16810593682568,174.995535575418));
#12256=CARTESIAN_POINT('Origin',(-54.5589537515075,2.89037996126418,174.712692862944));
#12257=CARTESIAN_POINT('Origin',(-54.7999573211759,4.14014685129092,175.985485069079));
#12258=CARTESIAN_POINT('Origin',(-54.1408102479648,0.722022427280349,175.985485069079));
#12259=CARTESIAN_POINT('',(-54.5335740892272,0.646282312434711,175.985485069079));
#12260=CARTESIAN_POINT('',(-54.5335740892272,0.646282312434712,175.985485069079));
#12261=CARTESIAN_POINT('',(-54.2726708967805,0.696594575640996,176.362269083675));
#12262=CARTESIAN_POINT('Origin',(-54.1408102479648,0.722022427280349,175.985485069079));
#12263=CARTESIAN_POINT('',(-54.0089495991491,0.747450278919701,175.608701054484));
#12264=CARTESIAN_POINT('Origin',(-54.1408102479648,0.722022427280349,175.985485069079));
#12265=CARTESIAN_POINT('Origin',(-54.1408102479648,0.722022427280349,175.985485069079));
#12266=CARTESIAN_POINT('Ctrl Pts',(-55.1161897096451,-2.27071607222657,
177.448351373365));
#12267=CARTESIAN_POINT('Ctrl Pts',(-55.0544324803005,-2.24407445661358,
177.516574922684));
#12268=CARTESIAN_POINT('Ctrl Pts',(-55.0031840696463,-2.2159075942787,177.564829510218));
#12269=CARTESIAN_POINT('Ctrl Pts',(-54.8981614763103,-2.14735807337978,
177.649345866972));
#12270=CARTESIAN_POINT('Ctrl Pts',(-54.848196955649,-2.10845499517373,177.68122338125));
#12271=CARTESIAN_POINT('Ctrl Pts',(-54.7062455015458,-1.97869616397794,
177.747598981208));
#12272=CARTESIAN_POINT('Ctrl Pts',(-54.6230552819493,-1.87505607340526,
177.751980177594));
#12273=CARTESIAN_POINT('Ctrl Pts',(-54.4781164600507,-1.64599936204779,
177.704020550018));
#12274=CARTESIAN_POINT('Ctrl Pts',(-54.4161687409529,-1.52036398038793,
177.652507519121));
#12275=CARTESIAN_POINT('Ctrl Pts',(-54.3240884061122,-1.31623292778147,
177.552502738263));
#12276=CARTESIAN_POINT('Ctrl Pts',(-54.2900300114527,-1.2450809441322,177.5168693343));
#12277=CARTESIAN_POINT('Ctrl Pts',(-54.2388806708887,-1.10092476185966,
177.429650782512));
#12278=CARTESIAN_POINT('Ctrl Pts',(-54.2230625419579,-1.02814126447079,
177.378422455576));
#12279=CARTESIAN_POINT('Ctrl Pts',(-54.1687570862725,-0.661100958902222,
177.107656526019));
#12280=CARTESIAN_POINT('Ctrl Pts',(-54.1632550913909,-0.344986943697024,
176.855601626641));
#12281=CARTESIAN_POINT('Ctrl Pts',(-54.1894883174704,0.100428951784895,
176.57062132681));
#12282=CARTESIAN_POINT('Ctrl Pts',(-54.2038650968969,0.243821813285216,
176.491645489995));
#12283=CARTESIAN_POINT('Ctrl Pts',(-54.2289503028814,0.435912884592043,
176.413053638658));
#12284=CARTESIAN_POINT('Ctrl Pts',(-54.2378694870404,0.495988408430007,
176.393461416067));
#12285=CARTESIAN_POINT('Ctrl Pts',(-54.2511575637744,0.57777536525398,176.374426535183));
#12286=CARTESIAN_POINT('Ctrl Pts',(-54.2555861991508,0.603644576350343,
176.369782059628));
#12287=CARTESIAN_POINT('Ctrl Pts',(-54.2642818917577,0.652365455860021,
176.363705099944));
#12288=CARTESIAN_POINT('Ctrl Pts',(-54.2669281652524,0.666814619551347,
176.362269083675));
#12289=CARTESIAN_POINT('Ctrl Pts',(-54.2726708967805,0.696594575640996,
176.362269083675));
#12290=CARTESIAN_POINT('Ctrl Pts',(-54.9611536226478,-1.61438316700751,
177.018013216499));
#12291=CARTESIAN_POINT('Ctrl Pts',(-54.9292844549615,-1.59689979741686,
177.061501366048));
#12292=CARTESIAN_POINT('Ctrl Pts',(-54.9347169869457,-1.59513306644644,
177.059466012753));
#12293=CARTESIAN_POINT('Ctrl Pts',(-54.9393829236175,-1.59207559169288,
177.070205982371));
#12294=CARTESIAN_POINT('Ctrl Pts',(-54.9521671405265,-1.59794122115585,
177.067981920184));
#12295=CARTESIAN_POINT('Ctrl Pts',(-55.0007420885566,-1.63157855374127,
177.067321317852));
#12296=CARTESIAN_POINT('Ctrl Pts',(-55.035179086296,-1.66960295600012,177.085015349648));
#12297=CARTESIAN_POINT('Ctrl Pts',(-55.0396054390644,-1.63669166623166,
177.119603765033));
#12298=CARTESIAN_POINT('Ctrl Pts',(-55.0210115508064,-1.57122240422777,
177.125346825549));
#12299=CARTESIAN_POINT('Ctrl Pts',(-54.9916258301057,-1.40601129473046,
177.119012727072));
#12300=CARTESIAN_POINT('Ctrl Pts',(-54.9808143890584,-1.33515491542406,
177.122292216748));
#12301=CARTESIAN_POINT('Ctrl Pts',(-54.95716312305,-1.20146912437994,177.090609934045));
#12302=CARTESIAN_POINT('Ctrl Pts',(-54.9459301778233,-1.14025139494389,
177.054154311007));
#12303=CARTESIAN_POINT('Ctrl Pts',(-54.9010485418089,-0.837221085805294,
176.830475957374));
#12304=CARTESIAN_POINT('Ctrl Pts',(-54.8933924651384,-0.543523047070829,
176.59567568837));
#12305=CARTESIAN_POINT('Ctrl Pts',(-54.9188659939004,-0.109419407590943,
176.317655840143));
#12306=CARTESIAN_POINT('Ctrl Pts',(-54.9330773739472,0.0346181647599921,
176.23753447689));
#12307=CARTESIAN_POINT('Ctrl Pts',(-54.9598081399055,0.239682185419695,
176.153510553493));
#12308=CARTESIAN_POINT('Ctrl Pts',(-54.9696067027056,0.306181698359097,
176.131488679163));
#12309=CARTESIAN_POINT('Ctrl Pts',(-54.985167831776,0.402075433542801,176.109129772912));
#12310=CARTESIAN_POINT('Ctrl Pts',(-54.9905018003277,0.433390482627809,
176.103410426781));
#12311=CARTESIAN_POINT('Ctrl Pts',(-55.0013966992521,0.494658609580997,
176.095691012754));
#12312=CARTESIAN_POINT('Ctrl Pts',(-55.0061011366799,0.520171112552638,
176.093689066957));
#12313=CARTESIAN_POINT('Ctrl Pts',(-55.012606581275,0.553906252953576,176.093689066957));
#12314=CARTESIAN_POINT('Ctrl Pts',(-54.3738267566562,-2.00237092626598,
176.637865020199));
#12315=CARTESIAN_POINT('Ctrl Pts',(-54.3525463517218,-1.98561856641678,
176.665739674622));
#12316=CARTESIAN_POINT('Ctrl Pts',(-54.3544769039845,-1.9794317280201,176.664843524849));
#12317=CARTESIAN_POINT('Ctrl Pts',(-54.3701639946021,-1.97656111293176,
176.660021126843));
#12318=CARTESIAN_POINT('Ctrl Pts',(-54.3898340629218,-1.98406009722412,
176.649873028566));
#12319=CARTESIAN_POINT('Ctrl Pts',(-54.4615150878692,-2.02680400188237,
176.627416363355));
#12320=CARTESIAN_POINT('Ctrl Pts',(-54.5129888400511,-2.0757703324506,176.634526145744));
#12321=CARTESIAN_POINT('Ctrl Pts',(-54.5552784049148,-2.06122690211322,
176.64442773024));
#12322=CARTESIAN_POINT('Ctrl Pts',(-54.5578076149692,-2.0038135240127,176.634785085717));
#12323=CARTESIAN_POINT('Ctrl Pts',(-54.5892177302657,-1.85411233048761,
176.591889300217));
#12324=CARTESIAN_POINT('Ctrl Pts',(-54.610530702465,-1.78996529622254,176.577740776828));
#12325=CARTESIAN_POINT('Ctrl Pts',(-54.6268123436843,-1.66507238716025,
176.528080652247));
#12326=CARTESIAN_POINT('Ctrl Pts',(-54.6208424301061,-1.60549754243094,
176.490359176158));
#12327=CARTESIAN_POINT('Ctrl Pts',(-54.5752745689856,-1.29850461246565,
176.263815183543));
#12328=CARTESIAN_POINT('Ctrl Pts',(-54.5643152196599,-0.983878310891091,
176.010083812441));
#12329=CARTESIAN_POINT('Ctrl Pts',(-54.5948528025329,-0.459382509277473,
175.674365954678));
#12330=CARTESIAN_POINT('Ctrl Pts',(-54.6123879900288,-0.274694122222572,
175.56925971577));
#12331=CARTESIAN_POINT('Ctrl Pts',(-54.6518354905867,0.0289042342998165,
175.444989413561));
#12332=CARTESIAN_POINT('Ctrl Pts',(-54.6672255747517,0.134792609497288,
175.409177545969));
#12333=CARTESIAN_POINT('Ctrl Pts',(-54.6945480274656,0.303452837912914,
175.369907772329));
#12334=CARTESIAN_POINT('Ctrl Pts',(-54.7043366789371,0.361315642399545,
175.359237745269));
#12335=CARTESIAN_POINT('Ctrl Pts',(-54.7254408307236,0.480524258303587,
175.344341053851));
#12336=CARTESIAN_POINT('Ctrl Pts',(-54.7391421008419,0.554236948300629,
175.340121037765));
#12337=CARTESIAN_POINT('Ctrl Pts',(-54.7488852836436,0.604761956232279,
175.340121037765));
#12338=CARTESIAN_POINT('Ctrl Pts',(-54.5288628436534,-2.65870383148503,
177.068203177065));
#12339=CARTESIAN_POINT('Ctrl Pts',(-54.4776943770608,-2.6327932256135,177.120813231257));
#12340=CARTESIAN_POINT('Ctrl Pts',(-54.4229439866851,-2.60020625585236,
177.170207022314));
#12341=CARTESIAN_POINT('Ctrl Pts',(-54.3289425472948,-2.53184359461866,
177.239161011444));
#12342=CARTESIAN_POINT('Ctrl Pts',(-54.2858638780443,-2.494573871242,177.263114489632));
#12343=CARTESIAN_POINT('Ctrl Pts',(-54.1670185008584,-2.37392161211904,
177.307694026711));
#12344=CARTESIAN_POINT('Ctrl Pts',(-54.1008650357044,-2.28122344985573,
177.30149097369));
#12345=CARTESIAN_POINT('Ctrl Pts',(-53.9937894259011,-2.07053459792936,
177.228844515225));
#12346=CARTESIAN_POINT('Ctrl Pts',(-53.9529648051158,-1.95295510017287,
177.161945779289));
#12347=CARTESIAN_POINT('Ctrl Pts',(-53.9216803062721,-1.76433396353862,
177.025379311408));
#12348=CARTESIAN_POINT('Ctrl Pts',(-53.9197463248593,-1.6998913249307,176.97231789438));
#12349=CARTESIAN_POINT('Ctrl Pts',(-53.9085298915231,-1.56452802463996,
176.867121500714));
#12350=CARTESIAN_POINT('Ctrl Pts',(-53.8979747942407,-1.4933874119578,176.814627320727));
#12351=CARTESIAN_POINT('Ctrl Pts',(-53.8429831134493,-1.12238448556273,
176.540995752188));
#12352=CARTESIAN_POINT('Ctrl Pts',(-53.8341778459125,-0.785342207517119,
176.270009750712));
#12353=CARTESIAN_POINT('Ctrl Pts',(-53.8654751261029,-0.249534149901716,
175.927331441344));
#12354=CARTESIAN_POINT('Ctrl Pts',(-53.8831757129786,-0.0654904736973553,
175.823370728875));
#12355=CARTESIAN_POINT('Ctrl Pts',(-53.9209776535626,0.225134933472168,
175.704532498726));
#12356=CARTESIAN_POINT('Ctrl Pts',(-53.9354883590865,0.324599319568198,
175.671150282872));
#12357=CARTESIAN_POINT('Ctrl Pts',(-53.960537759464,0.479152769624093,175.6352045346));
#12358=CARTESIAN_POINT('Ctrl Pts',(-53.9694210777602,0.531569736122078,
175.625609378116));
#12359=CARTESIAN_POINT('Ctrl Pts',(-53.9883260232292,0.638231104582612,
175.612355141042));
#12360=CARTESIAN_POINT('Ctrl Pts',(-53.9999691294144,0.700880455299337,
175.608701054484));
#12361=CARTESIAN_POINT('Ctrl Pts',(-54.0089495991491,0.747450278919698,
175.608701054484));
#12362=CARTESIAN_POINT('Ctrl Pts',(-54.6838989306507,-3.31503673670408,
177.498541333932));
#12363=CARTESIAN_POINT('Ctrl Pts',(-54.6028424023999,-3.27996788481022,
177.575886787893));
#12364=CARTESIAN_POINT('Ctrl Pts',(-54.4914110693857,-3.22098078368462,
177.675570519779));
#12365=CARTESIAN_POINT('Ctrl Pts',(-54.2877210999876,-3.08712607630556,
177.818300896045));
#12366=CARTESIAN_POINT('Ctrl Pts',(-54.1818936931668,-3.00508764525988,
177.876355950698));
#12367=CARTESIAN_POINT('Ctrl Pts',(-53.8725219138475,-2.7210392223557,177.987971690067));
#12368=CARTESIAN_POINT('Ctrl Pts',(-53.6887412313577,-2.48667656726087,
177.968455801636));
#12369=CARTESIAN_POINT('Ctrl Pts',(-53.4323004468874,-2.07984229374549,
177.81326130021));
#12370=CARTESIAN_POINT('Ctrl Pts',(-53.3481219952623,-1.90209667633303,
177.689106472861));
#12371=CARTESIAN_POINT('Ctrl Pts',(-53.2541428822785,-1.67455559658963,
177.4588693226));
#12372=CARTESIAN_POINT('Ctrl Pts',(-53.2289619472537,-1.60981735363885,
177.366895011932));
#12373=CARTESIAN_POINT('Ctrl Pts',(-53.1902474393619,-1.46398366211967,
177.206162349181));
#12374=CARTESIAN_POINT('Ctrl Pts',(-53.1751071583752,-1.38127728148465,
177.138895465296));
#12375=CARTESIAN_POINT('Ctrl Pts',(-53.1106916579129,-0.946264358659819,
176.818176320833));
#12376=CARTESIAN_POINT('Ctrl Pts',(-53.104040472165,-0.586806104143147,
176.529935688984));
#12377=CARTESIAN_POINT('Ctrl Pts',(-53.1360974496729,-0.0396857905259603,
176.18029692801));
#12378=CARTESIAN_POINT('Ctrl Pts',(-53.1539634359283,0.143713174827862,
176.077481741979));
#12379=CARTESIAN_POINT('Ctrl Pts',(-53.1901198165385,0.421365632644519,
175.964075583891));
#12380=CARTESIAN_POINT('Ctrl Pts',(-53.2037511434212,0.514406029639107,
175.933123019776));
#12381=CARTESIAN_POINT('Ctrl Pts',(-53.2265274914624,0.654852701335273,
175.900501296871));
#12382=CARTESIAN_POINT('Ctrl Pts',(-53.2345054765832,0.701823829844612,
175.891981010963));
#12383=CARTESIAN_POINT('Ctrl Pts',(-53.2512112157347,0.795937950861637,
175.880369228233));
#12384=CARTESIAN_POINT('Ctrl Pts',(-53.2607961579869,0.847523962298047,
175.877281071202));
#12385=CARTESIAN_POINT('Ctrl Pts',(-53.2690139146546,0.890138601607118,
175.877281071202));
#12386=CARTESIAN_POINT('Ctrl Pts',(-55.2712257966423,-2.92704897744562,
177.878689530232));
#12387=CARTESIAN_POINT('Ctrl Pts',(-55.1795805056396,-2.8912491158103,177.971648479319));
#12388=CARTESIAN_POINT('Ctrl Pts',(-55.071651152347,-2.83668212211097,178.070193007683));
#12389=CARTESIAN_POINT('Ctrl Pts',(-54.8569400290031,-2.70264055506668,
178.228485751573));
#12390=CARTESIAN_POINT('Ctrl Pts',(-54.7442267707714,-2.61896876919161,
178.294464842316));
#12391=CARTESIAN_POINT('Ctrl Pts',(-54.411748914535,-2.3258137742146,178.427876644564));
#12392=CARTESIAN_POINT('Ctrl Pts',(-54.2109314776027,-2.08050919081039,
178.41894500554));
#12393=CARTESIAN_POINT('Ctrl Pts',(-53.916627481037,-1.65530705786393,178.288437335003));
#12394=CARTESIAN_POINT('Ctrl Pts',(-53.8113259310995,-1.4695055565481,178.179668212693));
#12395=CARTESIAN_POINT('Ctrl Pts',(-53.6565509821185,-1.22645456083248,
177.985992749455));
#12396=CARTESIAN_POINT('Ctrl Pts',(-53.5992456338471,-1.15500697284035,
177.911446451852));
#12397=CARTESIAN_POINT('Ctrl Pts',(-53.5205982187275,-1.00038039933938,
177.768691630978));
#12398=CARTESIAN_POINT('Ctrl Pts',(-53.5001949060925,-0.916031133997679,
177.702690600146));
#12399=CARTESIAN_POINT('Ctrl Pts',(-53.4364656307362,-0.484980831999149,
177.384837094664));
#12400=CARTESIAN_POINT('Ctrl Pts',(-53.4331177176434,-0.146450840323217,
177.115527564913));
#12401=CARTESIAN_POINT('Ctrl Pts',(-53.4601106410404,0.310277311160734,
176.823586813476));
#12402=CARTESIAN_POINT('Ctrl Pts',(-53.4746528198466,0.453025461810439,
176.745756503099));
#12403=CARTESIAN_POINT('Ctrl Pts',(-53.4980924658573,0.632143583764391,
176.672596723823));
#12404=CARTESIAN_POINT('Ctrl Pts',(-53.5061322713752,0.685795118500917,
176.65543415297));
#12405=CARTESIAN_POINT('Ctrl Pts',(-53.5171472957729,0.75347529696516,176.639723297454));
#12406=CARTESIAN_POINT('Ctrl Pts',(-53.5206705979738,0.773898670072877,
176.636153692475));
#12407=CARTESIAN_POINT('Ctrl Pts',(-53.5271670842632,0.810072302139046,
176.631719187135));
#12408=CARTESIAN_POINT('Ctrl Pts',(-53.5277551938249,0.813458126550056,
176.630849100393));
#12409=CARTESIAN_POINT('Ctrl Pts',(-53.532735212286,0.839282898328416,176.630849100393));
#12410=CARTESIAN_POINT('Ctrl Pts',(-55.1161897096451,-2.27071607222657,
177.448351373365));
#12411=CARTESIAN_POINT('Ctrl Pts',(-55.0544324803005,-2.24407445661358,
177.516574922684));
#12412=CARTESIAN_POINT('Ctrl Pts',(-55.0031840696463,-2.2159075942787,177.564829510218));
#12413=CARTESIAN_POINT('Ctrl Pts',(-54.8981614763103,-2.14735807337978,
177.649345866972));
#12414=CARTESIAN_POINT('Ctrl Pts',(-54.848196955649,-2.10845499517373,177.68122338125));
#12415=CARTESIAN_POINT('Ctrl Pts',(-54.7062455015458,-1.97869616397794,
177.747598981208));
#12416=CARTESIAN_POINT('Ctrl Pts',(-54.6230552819493,-1.87505607340526,
177.751980177594));
#12417=CARTESIAN_POINT('Ctrl Pts',(-54.4781164600507,-1.64599936204779,
177.704020550018));
#12418=CARTESIAN_POINT('Ctrl Pts',(-54.4161687409529,-1.52036398038793,
177.652507519121));
#12419=CARTESIAN_POINT('Ctrl Pts',(-54.3240884061122,-1.31623292778147,
177.552502738263));
#12420=CARTESIAN_POINT('Ctrl Pts',(-54.2900300114527,-1.2450809441322,177.5168693343));
#12421=CARTESIAN_POINT('Ctrl Pts',(-54.2388806708887,-1.10092476185966,
177.429650782512));
#12422=CARTESIAN_POINT('Ctrl Pts',(-54.2230625419579,-1.02814126447079,
177.378422455576));
#12423=CARTESIAN_POINT('Ctrl Pts',(-54.1687570862725,-0.661100958902222,
177.107656526019));
#12424=CARTESIAN_POINT('Ctrl Pts',(-54.1632550913909,-0.344986943697024,
176.855601626641));
#12425=CARTESIAN_POINT('Ctrl Pts',(-54.1894883174704,0.100428951784895,
176.57062132681));
#12426=CARTESIAN_POINT('Ctrl Pts',(-54.2038650968969,0.243821813285216,
176.491645489995));
#12427=CARTESIAN_POINT('Ctrl Pts',(-54.2289503028814,0.435912884592043,
176.413053638658));
#12428=CARTESIAN_POINT('Ctrl Pts',(-54.2378694870404,0.495988408430007,
176.393461416067));
#12429=CARTESIAN_POINT('Ctrl Pts',(-54.2511575637744,0.57777536525398,176.374426535183));
#12430=CARTESIAN_POINT('Ctrl Pts',(-54.2555861991508,0.603644576350343,
176.369782059628));
#12431=CARTESIAN_POINT('Ctrl Pts',(-54.2642818917577,0.652365455860021,
176.363705099944));
#12432=CARTESIAN_POINT('Ctrl Pts',(-54.2669281652524,0.666814619551347,
176.362269083675));
#12433=CARTESIAN_POINT('Ctrl Pts',(-54.2726708967805,0.696594575640996,
176.362269083675));
#12434=CARTESIAN_POINT('',(-54.5288628436534,-2.65870383148502,177.068203177065));
#12435=CARTESIAN_POINT('',(-55.1161897096451,-2.27071607222657,177.448351373365));
#12436=CARTESIAN_POINT('Origin',(-54.8225262766493,-2.4647099518558,177.258277275215));
#12437=CARTESIAN_POINT('Ctrl Pts',(-54.5288628436534,-2.65870383148502,
177.068203177065));
#12438=CARTESIAN_POINT('Ctrl Pts',(-54.4776943770608,-2.6327932256135,177.120813231257));
#12439=CARTESIAN_POINT('Ctrl Pts',(-54.4229439866851,-2.60020625585236,
177.170207022314));
#12440=CARTESIAN_POINT('Ctrl Pts',(-54.3289425472948,-2.53184359461866,
177.239161011444));
#12441=CARTESIAN_POINT('Ctrl Pts',(-54.2858638780443,-2.494573871242,177.263114489632));
#12442=CARTESIAN_POINT('Ctrl Pts',(-54.1670185008584,-2.37392161211904,
177.307694026711));
#12443=CARTESIAN_POINT('Ctrl Pts',(-54.1008650357044,-2.28122344985573,
177.30149097369));
#12444=CARTESIAN_POINT('Ctrl Pts',(-53.9937894259011,-2.07053459792936,
177.228844515225));
#12445=CARTESIAN_POINT('Ctrl Pts',(-53.9529648051158,-1.95295510017287,
177.161945779289));
#12446=CARTESIAN_POINT('Ctrl Pts',(-53.9216803062721,-1.76433396353862,
177.025379311408));
#12447=CARTESIAN_POINT('Ctrl Pts',(-53.9197463248593,-1.6998913249307,176.97231789438));
#12448=CARTESIAN_POINT('Ctrl Pts',(-53.9085298915231,-1.56452802463996,
176.867121500714));
#12449=CARTESIAN_POINT('Ctrl Pts',(-53.8979747942407,-1.4933874119578,176.814627320727));
#12450=CARTESIAN_POINT('Ctrl Pts',(-53.8429831134493,-1.12238448556273,
176.540995752188));
#12451=CARTESIAN_POINT('Ctrl Pts',(-53.8341778459125,-0.785342207517119,
176.270009750712));
#12452=CARTESIAN_POINT('Ctrl Pts',(-53.8654751261029,-0.249534149901716,
175.927331441344));
#12453=CARTESIAN_POINT('Ctrl Pts',(-53.8831757129786,-0.0654904736973553,
175.823370728875));
#12454=CARTESIAN_POINT('Ctrl Pts',(-53.9209776535626,0.225134933472168,
175.704532498726));
#12455=CARTESIAN_POINT('Ctrl Pts',(-53.9354883590865,0.324599319568198,
175.671150282872));
#12456=CARTESIAN_POINT('Ctrl Pts',(-53.960537759464,0.479152769624093,175.6352045346));
#12457=CARTESIAN_POINT('Ctrl Pts',(-53.9694210777602,0.531569736122078,
175.625609378116));
#12458=CARTESIAN_POINT('Ctrl Pts',(-53.9883260232292,0.638231104582612,
175.612355141042));
#12459=CARTESIAN_POINT('Ctrl Pts',(-53.9999691294144,0.700880455299337,
175.608701054484));
#12460=CARTESIAN_POINT('Ctrl Pts',(-54.0089495991491,0.747450278919701,
175.608701054484));
#12461=CARTESIAN_POINT('Ctrl Pts',(-55.1161897096451,-2.27071607222657,
177.448351373365));
#12462=CARTESIAN_POINT('Ctrl Pts',(-55.0544324803005,-2.24407445661358,
177.516574922684));
#12463=CARTESIAN_POINT('Ctrl Pts',(-55.0031840696463,-2.2159075942787,177.564829510218));
#12464=CARTESIAN_POINT('Ctrl Pts',(-54.8981614763103,-2.14735807337978,
177.649345866972));
#12465=CARTESIAN_POINT('Ctrl Pts',(-54.848196955649,-2.10845499517373,177.68122338125));
#12466=CARTESIAN_POINT('Ctrl Pts',(-54.7062455015458,-1.97869616397794,
177.747598981208));
#12467=CARTESIAN_POINT('Ctrl Pts',(-54.6230552819493,-1.87505607340526,
177.751980177594));
#12468=CARTESIAN_POINT('Ctrl Pts',(-54.4781164600507,-1.64599936204779,
177.704020550018));
#12469=CARTESIAN_POINT('Ctrl Pts',(-54.4161687409529,-1.52036398038793,
177.652507519121));
#12470=CARTESIAN_POINT('Ctrl Pts',(-54.3240884061122,-1.31623292778147,
177.552502738263));
#12471=CARTESIAN_POINT('Ctrl Pts',(-54.2900300114527,-1.2450809441322,177.5168693343));
#12472=CARTESIAN_POINT('Ctrl Pts',(-54.2388806708887,-1.10092476185966,
177.429650782512));
#12473=CARTESIAN_POINT('Ctrl Pts',(-54.2230625419579,-1.02814126447079,
177.378422455576));
#12474=CARTESIAN_POINT('Ctrl Pts',(-54.1687570862725,-0.661100958902222,
177.107656526019));
#12475=CARTESIAN_POINT('Ctrl Pts',(-54.1632550913909,-0.344986943697024,
176.855601626641));
#12476=CARTESIAN_POINT('Ctrl Pts',(-54.1894883174704,0.100428951784895,
176.57062132681));
#12477=CARTESIAN_POINT('Ctrl Pts',(-54.2038650968969,0.243821813285216,
176.491645489995));
#12478=CARTESIAN_POINT('Ctrl Pts',(-54.2289503028814,0.435912884592043,
176.413053638658));
#12479=CARTESIAN_POINT('Ctrl Pts',(-54.2378694870404,0.495988408430007,
176.393461416067));
#12480=CARTESIAN_POINT('Ctrl Pts',(-54.2511575637744,0.57777536525398,176.374426535183));
#12481=CARTESIAN_POINT('Ctrl Pts',(-54.2555861991508,0.603644576350343,
176.369782059628));
#12482=CARTESIAN_POINT('Ctrl Pts',(-54.2642818917577,0.652365455860021,
176.363705099944));
#12483=CARTESIAN_POINT('Ctrl Pts',(-54.2669281652524,0.666814619551347,
176.362269083675));
#12484=CARTESIAN_POINT('Ctrl Pts',(-54.2726708967805,0.696594575640996,
176.362269083675));
#12485=CARTESIAN_POINT('Ctrl Pts',(-50.193114320713,-27.8005016688432,177.448440461337));
#12486=CARTESIAN_POINT('Ctrl Pts',(-50.1356777281885,-27.7780416249781,
177.514251363723));
#12487=CARTESIAN_POINT('Ctrl Pts',(-50.0768656935625,-27.751543311514,177.569181845458));
#12488=CARTESIAN_POINT('Ctrl Pts',(-49.9502510673185,-27.7006718917524,
177.678131488152));
#12489=CARTESIAN_POINT('Ctrl Pts',(-49.8836384545372,-27.6746069642733,
177.728584647058));
#12490=CARTESIAN_POINT('Ctrl Pts',(-49.6751767137455,-27.5945945456976,
177.866776279515));
#12491=CARTESIAN_POINT('Ctrl Pts',(-49.5241175159801,-27.5384622401806,
177.941191651987));
#12492=CARTESIAN_POINT('Ctrl Pts',(-49.052722448706,-27.3677108924734,178.102046365205));
#12493=CARTESIAN_POINT('Ctrl Pts',(-48.713006227557,-27.2491092781452,178.126053652285));
#12494=CARTESIAN_POINT('Ctrl Pts',(-47.7382795874562,-26.9019657740439,
177.942209528285));
#12495=CARTESIAN_POINT('Ctrl Pts',(-47.1597470877608,-26.6842880122364,
177.461567693823));
#12496=CARTESIAN_POINT('Ctrl Pts',(-46.658904710499,-26.3725604903201,176.179580952166));
#12497=CARTESIAN_POINT('Ctrl Pts',(-46.744016732095,-26.2835354545934,175.410971277798));
#12498=CARTESIAN_POINT('Ctrl Pts',(-47.5354179070377,-26.2224078706935,
174.242909311213));
#12499=CARTESIAN_POINT('Ctrl Pts',(-48.2245449656354,-26.2493771368743,
173.87343933243));
#12500=CARTESIAN_POINT('Ctrl Pts',(-49.6317089464608,-26.3060463238627,
173.871895146128));
#12501=CARTESIAN_POINT('Ctrl Pts',(-50.3230600395606,-26.332977077053,174.238655026377));
#12502=CARTESIAN_POINT('Ctrl Pts',(-51.1153496063116,-26.2743348509258,
175.387691644257));
#12503=CARTESIAN_POINT('Ctrl Pts',(-51.2096393582444,-26.1855070701005,
176.164686974611));
#12504=CARTESIAN_POINT('Ctrl Pts',(-50.7213268039385,-25.8775623946772,
177.442968877094));
#12505=CARTESIAN_POINT('Ctrl Pts',(-50.1473617008829,-25.6602454668112,
177.932812658479));
#12506=CARTESIAN_POINT('Ctrl Pts',(-48.8451246534299,-25.1962898596545,
178.190564242377));
#12507=CARTESIAN_POINT('Ctrl Pts',(-48.1356293396501,-24.9529458243571,
177.955714348281));
#12508=CARTESIAN_POINT('Ctrl Pts',(-47.2268076672755,-24.5631416907191,
176.954286183848));
#12509=CARTESIAN_POINT('Ctrl Pts',(-47.0395646158613,-24.4209960169422,
176.20954077848));
#12510=CARTESIAN_POINT('Ctrl Pts',(-47.370313215787,-24.2726666068476,174.855768290097));
#12511=CARTESIAN_POINT('Ctrl Pts',(-47.8845545017147,-24.265674947158,174.26583855031));
#12512=CARTESIAN_POINT('Ctrl Pts',(-49.1994460468846,-24.3046603227726,
173.764180115318));
#12513=CARTESIAN_POINT('Ctrl Pts',(-49.9762257647407,-24.3480555327739,
173.861039734223));
#12514=CARTESIAN_POINT('Ctrl Pts',(-51.1285193941288,-24.3574791486806,
174.66646218052));
#12515=CARTESIAN_POINT('Ctrl Pts',(-51.4882290443068,-24.3203491702665,
175.364132112564));
#12516=CARTESIAN_POINT('Ctrl Pts',(-51.4777341832408,-24.1036300286494,
176.755680066459));
#12517=CARTESIAN_POINT('Ctrl Pts',(-51.1141102527119,-23.9275319100486,
177.423612084264));
#12518=CARTESIAN_POINT('Ctrl Pts',(-49.9940329966114,-23.4994535030053,
178.148719290634));
#12519=CARTESIAN_POINT('Ctrl Pts',(-49.2531996565364,-23.2503850964097,
178.195074921104));
#12520=CARTESIAN_POINT('Ctrl Pts',(-48.0540724826088,-22.804580182732,177.607487959387));
#12521=CARTESIAN_POINT('Ctrl Pts',(-47.6174629086983,-22.6140260251447,
176.985139741962));
#12522=CARTESIAN_POINT('Ctrl Pts',(-47.4549919432363,-22.3698803060775,
175.609945370482));
#12523=CARTESIAN_POINT('Ctrl Pts',(-47.7329522193418,-22.3169255939418,
174.876470615888));
#12524=CARTESIAN_POINT('Ctrl Pts',(-48.8440385240951,-22.3059754149369,
173.902867041218));
#12525=CARTESIAN_POINT('Ctrl Pts',(-49.7035599970344,-22.3554674780819,
173.739637329099));
#12526=CARTESIAN_POINT('Ctrl Pts',(-51.1531706356154,-22.4011313967338,
174.265066374312));
#12527=CARTESIAN_POINT('Ctrl Pts',(-51.7115054154064,-22.3910761212842,
174.945624054023));
#12528=CARTESIAN_POINT('Ctrl Pts',(-51.9563259347572,-22.2045289991918,
176.459132103654));
#12529=CARTESIAN_POINT('Ctrl Pts',(-51.63765119649,-22.0251559400258,177.262331468575));
#12530=CARTESIAN_POINT('Ctrl Pts',(-50.4571461815608,-21.5627984935069,
178.149907937338));
#12531=CARTESIAN_POINT('Ctrl Pts',(-49.6222512854117,-21.2849471395443,
178.217719280236));
#12532=CARTESIAN_POINT('Ctrl Pts',(-48.3256452005116,-20.7988977065915,
177.525255091295));
#12533=CARTESIAN_POINT('Ctrl Pts',(-47.8935170509031,-20.5993012814682,
176.78942555283));
#12534=CARTESIAN_POINT('Ctrl Pts',(-47.9069259765589,-20.3679964193449,
175.264267840625));
#12535=CARTESIAN_POINT('Ctrl Pts',(-48.3565963500671,-20.33698501403,174.508050023486));
#12536=CARTESIAN_POINT('Ctrl Pts',(-49.7115395236169,-20.3645147337819,
173.767258025586));
#12537=CARTESIAN_POINT('Ctrl Pts',(-50.5919963646361,-20.4163759449694,
173.798730113887));
#12538=CARTESIAN_POINT('Ctrl Pts',(-51.8921615926268,-20.4324111199544,
174.637786957993));
#12539=CARTESIAN_POINT('Ctrl Pts',(-52.2870845316673,-20.391715494119,175.425932171935));
#12540=CARTESIAN_POINT('Ctrl Pts',(-52.1845249551972,-20.1359343420921,
176.949348485014));
#12541=CARTESIAN_POINT('Ctrl Pts',(-51.6978717551623,-19.9258306519252,
177.647217385389));
#12542=CARTESIAN_POINT('Ctrl Pts',(-50.3567743114224,-19.4332812849397,
178.229888643815));
#12543=CARTESIAN_POINT('Ctrl Pts',(-49.531482093434,-19.1564117811874,178.098575810452));
#12544=CARTESIAN_POINT('Ctrl Pts',(-48.4209526978951,-18.7085233315365,
177.123331466978));
#12545=CARTESIAN_POINT('Ctrl Pts',(-48.1597795720535,-18.5402167412103,
176.29718764283));
#12546=CARTESIAN_POINT('Ctrl Pts',(-48.5145782694716,-18.3739619700934,
174.800216258582));
#12547=CARTESIAN_POINT('Ctrl Pts',(-49.1216168980297,-18.3741927637648,
174.159897255644));
#12548=CARTESIAN_POINT('Ctrl Pts',(-50.6124880467131,-18.4256628314289,
173.74530968569));
#12549=CARTESIAN_POINT('Ctrl Pts',(-51.4570089590119,-18.472296203581,173.973986288395));
#12550=CARTESIAN_POINT('Ctrl Pts',(-52.5367755134872,-18.4465314340497,
175.076321400051));
#12551=CARTESIAN_POINT('Ctrl Pts',(-52.7461464663159,-18.3691716102472,
175.928004990245));
#12552=CARTESIAN_POINT('Ctrl Pts',(-52.3166330239091,-18.0526500335514,
177.376965544067));
#12553=CARTESIAN_POINT('Ctrl Pts',(-51.6857211698905,-17.8130496454,177.945754508989));
#12554=CARTESIAN_POINT('Ctrl Pts',(-50.2465394893753,-17.3007990625156,
178.194297846636));
#12555=CARTESIAN_POINT('Ctrl Pts',(-49.4703000985441,-17.0343670318334,
177.871754882023));
#12556=CARTESIAN_POINT('Ctrl Pts',(-48.6088763818932,-16.6321365971318,
176.648991214725));
#12557=CARTESIAN_POINT('Ctrl Pts',(-48.5409020769561,-16.5028432711256,
175.78526591443));
#12558=CARTESIAN_POINT('Ctrl Pts',(-49.2164515058916,-16.3991203888251,
174.401518908745));
#12559=CARTESIAN_POINT('Ctrl Pts',(-49.9496118192587,-16.4227354715302,
173.914202886417));
#12560=CARTESIAN_POINT('Ctrl Pts',(-51.4902606534728,-16.4861638259448,
173.836744887307));
#12561=CARTESIAN_POINT('Ctrl Pts',(-52.2697075969923,-16.5185243960147,
174.249627738192));
#12562=CARTESIAN_POINT('Ctrl Pts',(-53.0792623986938,-16.4399376212412,
175.566241461313));
#12563=CARTESIAN_POINT('Ctrl Pts',(-53.0958608617722,-16.3264383488088,
176.440260240546));
#12564=CARTESIAN_POINT('Ctrl Pts',(-52.3498924896565,-15.9464100326616,
177.743856795072));
#12565=CARTESIAN_POINT('Ctrl Pts',(-51.6136771994172,-15.6882407493956,
178.142477224647));
#12566=CARTESIAN_POINT('Ctrl Pts',(-50.1619939854693,-15.1743526813971,
178.045393567771));
#12567=CARTESIAN_POINT('Ctrl Pts',(-49.479535393056,-14.9249532161513,177.547481856475));
#12568=CARTESIAN_POINT('Ctrl Pts',(-48.9083003859244,-14.5811172796918,
176.154888290848));
#12569=CARTESIAN_POINT('Ctrl Pts',(-49.032687325759,-14.4872017268269,175.286386043965));
#12570=CARTESIAN_POINT('Ctrl Pts',(-50.002899927607,-14.4395306566209,174.08106638639));
#12571=CARTESIAN_POINT('Ctrl Pts',(-50.8258619899905,-14.4815667576624,
173.768688449528));
#12572=CARTESIAN_POINT('Ctrl Pts',(-52.3490472247602,-14.5391579602322,
174.044477097964));
#12573=CARTESIAN_POINT('Ctrl Pts',(-53.0108480437211,-14.5505369630929,
174.618897762295));
#12574=CARTESIAN_POINT('Ctrl Pts',(-53.508606726061,-14.41258118913,176.072854784516));
#12575=CARTESIAN_POINT('Ctrl Pts',(-53.3308496256547,-14.2605010523332,
176.92211652172));
#12576=CARTESIAN_POINT('Ctrl Pts',(-52.3234046589676,-13.8325238003689,
178.011250192421));
#12577=CARTESIAN_POINT('Ctrl Pts',(-51.5138129382755,-13.5585438056648,
178.229366209696));
#12578=CARTESIAN_POINT('Ctrl Pts',(-50.1182607249297,-13.0546721198729,
177.788098654291));
#12579=CARTESIAN_POINT('Ctrl Pts',(-49.5630188185408,-12.8308644828691,
177.140857971114));
#12580=CARTESIAN_POINT('Ctrl Pts',(-49.3219040202974,-12.5483689245281,
175.637957478437));
#12581=CARTESIAN_POINT('Ctrl Pts',(-49.6365594730894,-12.4926951709364,
174.821179942866));
#12582=CARTESIAN_POINT('Ctrl Pts',(-50.8450351424658,-12.4918253386163,
173.862170041067));
#12583=CARTESIAN_POINT('Ctrl Pts',(-51.7160671936879,-12.5420406725331,
173.742988789581));
#12584=CARTESIAN_POINT('Ctrl Pts',(-53.1380531234061,-12.5824907099911,
174.344563971126));
#12585=CARTESIAN_POINT('Ctrl Pts',(-53.661497991413,-12.565516429584,175.054752397452));
#12586=CARTESIAN_POINT('Ctrl Pts',(-53.8242077932451,-12.3622912981454,
176.579637740953));
#12587=CARTESIAN_POINT('Ctrl Pts',(-53.4635573374974,-12.1759538811977,
177.362604506387));
#12588=CARTESIAN_POINT('Ctrl Pts',(-52.2358756182636,-11.7031645393402,
178.179207046235));
#12589=CARTESIAN_POINT('Ctrl Pts',(-51.404471480006,-11.4266005921062,178.198059647233));
#12590=CARTESIAN_POINT('Ctrl Pts',(-50.1465877134854,-10.9499764840513,
177.440684540534));
#12591=CARTESIAN_POINT('Ctrl Pts',(-49.7512566691313,-10.7559713173261,
176.677961727673));
#12592=CARTESIAN_POINT('Ctrl Pts',(-49.8442980389787,-10.5402489724976,
175.152069846099));
#12593=CARTESIAN_POINT('Ctrl Pts',(-50.3336227209985,-10.5166703329192,
174.417963751365));
#12594=CARTESIAN_POINT('Ctrl Pts',(-51.729412313951,-10.5511670115394,173.750914008412));
#12595=CARTESIAN_POINT('Ctrl Pts',(-52.6055357660183,-10.6034581645062,
173.829125569603));
#12596=CARTESIAN_POINT('Ctrl Pts',(-53.8591972775733,-10.6090268187652,
174.739479897504));
#12597=CARTESIAN_POINT('Ctrl Pts',(-54.2075655427863,-10.559958422732,175.542285446703));
#12598=CARTESIAN_POINT('Ctrl Pts',(-54.0309723767407,-10.2919570312328,
177.05153449857));
#12599=CARTESIAN_POINT('Ctrl Pts',(-53.5065211660476,-10.0729835636969,
177.724885949439));
#12600=CARTESIAN_POINT('Ctrl Pts',(-52.1359327706082,-9.57501150980407,
178.231990439602));
#12601=CARTESIAN_POINT('Ctrl Pts',(-51.3168725161042,-9.29919601638729,
178.055337178134));
#12602=CARTESIAN_POINT('Ctrl Pts',(-50.258716477129,-8.86039345968628,177.014257444883));
#12603=CARTESIAN_POINT('Ctrl Pts',(-50.0419858596938,-8.70190296068798,
176.174822144773));
#12604=CARTESIAN_POINT('Ctrl Pts',(-50.4788136762356,-8.55014763089762,
174.697436550109));
#12605=CARTESIAN_POINT('Ctrl Pts',(-51.1165600370436,-8.55674976323144,
174.095019459488));
#12606=CARTESIAN_POINT('Ctrl Pts',(-52.6206590619166,-8.6128620697194,173.755704628284));
#12607=CARTESIAN_POINT('Ctrl Pts',(-53.456626592603,-8.65630954771657,174.029197443714));
#12608=CARTESIAN_POINT('Ctrl Pts',(-54.4781193003427,-8.6195332279715,175.187078119489));
#12609=CARTESIAN_POINT('Ctrl Pts',(-54.643602443466,-8.53353572012608,176.04949882023));
#12610=CARTESIAN_POINT('Ctrl Pts',(-54.1354947853707,-8.20096498746117,
177.472181687833));
#12611=CARTESIAN_POINT('Ctrl Pts',(-53.4760203027823,-7.95706608118669,
178.003825172765));
#12612=CARTESIAN_POINT('Ctrl Pts',(-52.0249165538012,-7.441132564782,178.167825277993));
#12613=CARTESIAN_POINT('Ctrl Pts',(-51.2723007652614,-7.17976116760829,
177.802466009854));
#12614=CARTESIAN_POINT('Ctrl Pts',(-50.4742318046734,-6.79179686888332,
176.539214575509));
#12615=CARTESIAN_POINT('Ctrl Pts',(-50.4508393849021,-6.66952799804251,
175.667365550039));
#12616=CARTESIAN_POINT('Ctrl Pts',(-51.1982775200671,-6.57992894303025,
174.318931761547));
#12617=CARTESIAN_POINT('Ctrl Pts',(-51.9567203354133,-6.60831910752051,
173.869388776842));
#12618=CARTESIAN_POINT('Ctrl Pts',(-53.5030461170827,-6.67180659392302,
173.876188814802));
#12619=CARTESIAN_POINT('Ctrl Pts',(-54.2579318048227,-6.70074853854407,
174.329266762268));
#12620=CARTESIAN_POINT('Ctrl Pts',(-54.9950541895712,-6.6067812144727,175.688231083653));
#12621=CARTESIAN_POINT('Ctrl Pts',(-54.9633937640365,-6.48434226598442,
176.556150922255));
#12622=CARTESIAN_POINT('Ctrl Pts',(-54.1573516980127,-6.0949735677162,177.812809342709));
#12623=CARTESIAN_POINT('Ctrl Pts',(-53.3979887985791,-5.83073710308303,
178.172806822259));
#12624=CARTESIAN_POINT('Ctrl Pts',(-51.9519097716579,-5.31810666795101,
177.994568269632));
#12625=CARTESIAN_POINT('Ctrl Pts',(-51.2952074816856,-5.0735953089356,177.458800517348));
#12626=CARTESIAN_POINT('Ctrl Pts',(-50.7993635736617,-4.74342220821161,
176.031468409862));
#12627=CARTESIAN_POINT('Ctrl Pts',(-50.9692613848378,-4.65940397939939,
175.170313217647));
#12628=CARTESIAN_POINT('Ctrl Pts',(-52.0040245669764,-4.62293999106357,
174.01934301833));
#12629=CARTESIAN_POINT('Ctrl Pts',(-52.8385688131003,-4.66759138415716,
173.754231358386));
#12630=CARTESIAN_POINT('Ctrl Pts',(-54.3414847379305,-4.72329909029368,
174.103969484305));
#12631=CARTESIAN_POINT('Ctrl Pts',(-54.9761466933045,-4.72791014175074,
174.714716972292));
#12632=CARTESIAN_POINT('Ctrl Pts',(-55.3975165431988,-4.57549651155636,
176.192173272167));
#12633=CARTESIAN_POINT('Ctrl Pts',(-55.1760506072609,-4.4148786220368,177.03103539143));
#12634=CARTESIAN_POINT('Ctrl Pts',(-54.1093043232961,-3.97451188101218,
178.061753391873));
#12635=CARTESIAN_POINT('Ctrl Pts',(-53.2902925544343,-3.69995792969149,
178.233822626392));
#12636=CARTESIAN_POINT('Ctrl Pts',(-51.9203920380846,-3.19963469730891,
177.711493690972));
#12637=CARTESIAN_POINT('Ctrl Pts',(-51.4044324721558,-2.98383265912278,
177.036002564632));
#12638=CARTESIAN_POINT('Ctrl Pts',(-51.237949425703,-2.71774512370317,175.525044339462));
#12639=CARTESIAN_POINT('Ctrl Pts',(-51.5957499271559,-2.66894330374766,
174.721509320474));
#12640=CARTESIAN_POINT('Ctrl Pts',(-52.8541051305037,-2.67783999801612,
173.825937213487));
#12641=CARTESIAN_POINT('Ctrl Pts',(-53.7315999697276,-2.7292086653859,173.7525048498));
#12642=CARTESIAN_POINT('Ctrl Pts',(-55.1208667949195,-2.76252327401043,
174.431246184642));
#12643=CARTESIAN_POINT('Ctrl Pts',(-55.6054709668258,-2.73893798071373,
175.167402226862));
#12644=CARTESIAN_POINT('Ctrl Pts',(-55.6603171863937,-2.58869274068622,
176.211840888345));
#12645=CARTESIAN_POINT('Ctrl Pts',(-55.6210463302226,-2.5392081864434,176.490448482462));
#12646=CARTESIAN_POINT('Ctrl Pts',(-55.4836397365907,-2.4479441182576,176.880586390838));
#12647=CARTESIAN_POINT('Ctrl Pts',(-55.4253285390117,-2.41535251334816,
177.005027857449));
#12648=CARTESIAN_POINT('Ctrl Pts',(-55.321414213033,-2.36345060131236,177.180440236558));
#12649=CARTESIAN_POINT('Ctrl Pts',(-55.2840225057543,-2.34563722905757,
177.23703696138));
#12650=CARTESIAN_POINT('Ctrl Pts',(-55.2039936793606,-2.30896761153951,
177.345998347345));
#12651=CARTESIAN_POINT('Ctrl Pts',(-55.1587206712145,-2.28906361698866,
177.401367187303));
#12652=CARTESIAN_POINT('Ctrl Pts',(-55.1161897096451,-2.27071607222657,
177.448351373365));
#12653=CARTESIAN_POINT('Ctrl Pts',(-50.0383214665825,-27.1440081492037,
177.018259765604));
#12654=CARTESIAN_POINT('Ctrl Pts',(-49.9984978891038,-27.1200869921306,
177.079962725598));
#12655=CARTESIAN_POINT('Ctrl Pts',(-49.9575055461974,-27.1020674615118,
177.117111982701));
#12656=CARTESIAN_POINT('Ctrl Pts',(-49.8677888002033,-27.0582153119246,
177.208150208202));
#12657=CARTESIAN_POINT('Ctrl Pts',(-49.8200811333233,-27.0356913176731,
177.250904604008));
#12658=CARTESIAN_POINT('Ctrl Pts',(-49.6696339972988,-26.9667169890279,
177.369319858048));
#12659=CARTESIAN_POINT('Ctrl Pts',(-49.5596041625372,-26.9190141211719,
177.434440092329));
#12660=CARTESIAN_POINT('Ctrl Pts',(-49.2118492777513,-26.7720570333375,
177.585359994682));
#12661=CARTESIAN_POINT('Ctrl Pts',(-48.9561313182544,-26.6696252716912,
177.624018992736));
#12662=CARTESIAN_POINT('Ctrl Pts',(-48.2061347626312,-26.3651189875991,
177.541325063495));
#12663=CARTESIAN_POINT('Ctrl Pts',(-47.7414452899411,-26.1688071749961,
177.206816180124));
#12664=CARTESIAN_POINT('Ctrl Pts',(-47.2997616792461,-25.8707230428421,
176.259912393579));
#12665=CARTESIAN_POINT('Ctrl Pts',(-47.3254088075791,-25.7696878441865,
175.668385446485));
#12666=CARTESIAN_POINT('Ctrl Pts',(-47.8755348089008,-25.6608852645148,
174.730075629747));
#12667=CARTESIAN_POINT('Ctrl Pts',(-48.3883745667453,-25.6533154874374,
174.409130171609));
#12668=CARTESIAN_POINT('Ctrl Pts',(-49.4697935970405,-25.6493947609597,
174.331547147859));
#12669=CARTESIAN_POINT('Ctrl Pts',(-50.0242338430418,-25.649381701477,174.571983854445));
#12670=CARTESIAN_POINT('Ctrl Pts',(-50.7048786270563,-25.5680766842178,
175.408205503607));
#12671=CARTESIAN_POINT('Ctrl Pts',(-50.8241348799264,-25.4835527568238,
175.999504945815));
#12672=CARTESIAN_POINT('Ctrl Pts',(-50.5299373615978,-25.2151761375736,
177.003363164347));
#12673=CARTESIAN_POINT('Ctrl Pts',(-50.1239438073276,-25.0297634587285,
177.413176265946));
#12674=CARTESIAN_POINT('Ctrl Pts',(-49.1505246752548,-24.6280758402134,
177.688626402201));
#12675=CARTESIAN_POINT('Ctrl Pts',(-48.5986534337901,-24.4145815428545,
177.549736774231));
#12676=CARTESIAN_POINT('Ctrl Pts',(-47.8611459428243,-24.0600384609719,
176.839550282587));
#12677=CARTESIAN_POINT('Ctrl Pts',(-47.6799485846058,-23.9185188665616,
176.282427966132));
#12678=CARTESIAN_POINT('Ctrl Pts',(-47.8667875018081,-23.7413010936383,
175.228664295839));
#12679=CARTESIAN_POINT('Ctrl Pts',(-48.2335406641398,-23.7053609783786,
174.748651320702));
#12680=CARTESIAN_POINT('Ctrl Pts',(-49.2178139490401,-23.6827183215843,
174.294936194443));
#12681=CARTESIAN_POINT('Ctrl Pts',(-49.8219962257384,-23.6923479099038,
174.323992647469));
#12682=CARTESIAN_POINT('Ctrl Pts',(-50.7591498572879,-23.6591435932359,
174.876124371948));
#12683=CARTESIAN_POINT('Ctrl Pts',(-51.077522753783,-23.6134950148359,175.39172485521));
#12684=CARTESIAN_POINT('Ctrl Pts',(-51.1535820381579,-23.415693423287,176.455061557909));
#12685=CARTESIAN_POINT('Ctrl Pts',(-50.918643706726,-23.2638702537623,176.988610346676));
#12686=CARTESIAN_POINT('Ctrl Pts',(-50.1109113395739,-22.8948872174005,
177.611393006538));
#12687=CARTESIAN_POINT('Ctrl Pts',(-49.550353441179,-22.680074585543,177.689808241912));
#12688=CARTESIAN_POINT('Ctrl Pts',(-48.6137447048011,-22.28702457331,177.311258226648));
#12689=CARTESIAN_POINT('Ctrl Pts',(-48.2490117887893,-22.1098470443037,
176.862573175931));
#12690=CARTESIAN_POINT('Ctrl Pts',(-48.0569364843034,-21.8588516971627,
175.821098220226));
#12691=CARTESIAN_POINT('Ctrl Pts',(-48.2348449020816,-21.7860567828884,
175.244332219005));
#12692=CARTESIAN_POINT('Ctrl Pts',(-49.0386897150743,-21.7181941257994,
174.442583421401));
#12693=CARTESIAN_POINT('Ctrl Pts',(-49.6927278496366,-21.7268807239962,
174.267611662058));
#12694=CARTESIAN_POINT('Ctrl Pts',(-50.8411043798997,-21.7141199241716,
174.588524908528));
#12695=CARTESIAN_POINT('Ctrl Pts',(-51.3094013702521,-21.6876269507243,
175.077312328235));
#12696=CARTESIAN_POINT('Ctrl Pts',(-51.5921855585383,-21.5071481278118,
176.224756535618));
#12697=CARTESIAN_POINT('Ctrl Pts',(-51.3974806497779,-21.3525654190584,
176.857134695111));
#12698=CARTESIAN_POINT('Ctrl Pts',(-50.5541169969121,-20.9549536496367,
177.606432421015));
#12699=CARTESIAN_POINT('Ctrl Pts',(-49.9226700094089,-20.7151144402318,
177.707627413831));
#12700=CARTESIAN_POINT('Ctrl Pts',(-48.9071810235129,-20.2857229365746,
177.254800594979));
#12701=CARTESIAN_POINT('Ctrl Pts',(-48.539258060867,-20.0973264562627,176.718436772752));
#12702=CARTESIAN_POINT('Ctrl Pts',(-48.475069365768,-19.8507243142978,175.553477519371));
#12703=CARTESIAN_POINT('Ctrl Pts',(-48.7817617425817,-19.793065331538,174.952184411851));
#12704=CARTESIAN_POINT('Ctrl Pts',(-49.7883433018784,-19.7521647995451,
174.308551222089));
#12705=CARTESIAN_POINT('Ctrl Pts',(-50.4672686416896,-19.7660480884512,
174.284275257332));
#12706=CARTESIAN_POINT('Ctrl Pts',(-51.5185621567429,-19.7338211938064,
174.853733695028));
#12707=CARTESIAN_POINT('Ctrl Pts',(-51.8704305933054,-19.6836035315617,
175.436932234299));
#12708=CARTESIAN_POINT('Ctrl Pts',(-51.8843323266907,-19.4527281797322,
176.606134032902));
#12709=CARTESIAN_POINT('Ctrl Pts',(-51.5571193795133,-19.2721887380014,
177.170821269618));
#12710=CARTESIAN_POINT('Ctrl Pts',(-50.5738822832083,-18.8483164964054,
177.696322750616));
#12711=CARTESIAN_POINT('Ctrl Pts',(-49.9420101663495,-18.6096692642048,
177.644259926591));
#12712=CARTESIAN_POINT('Ctrl Pts',(-49.0472024681392,-18.2021277928874,
176.964465534643));
#12713=CARTESIAN_POINT('Ctrl Pts',(-48.8080140865945,-18.0389468515475,
176.349664596734));
#12714=CARTESIAN_POINT('Ctrl Pts',(-49.0066488397389,-17.8423059144124,
175.186793179499));
#12715=CARTESIAN_POINT('Ctrl Pts',(-49.4421820059815,-17.8082452535064,
174.661978305101));
#12716=CARTESIAN_POINT('Ctrl Pts',(-50.56604357313,-17.7913894148755,174.265152819574));
#12717=CARTESIAN_POINT('Ctrl Pts',(-51.2311395254822,-17.8022399917982,
174.391161445375));
#12718=CARTESIAN_POINT('Ctrl Pts',(-52.1286453083844,-17.7409968363402,
175.174698745784));
#12719=CARTESIAN_POINT('Ctrl Pts',(-52.340061283037,-17.6649540872478,175.813880719354));
#12720=CARTESIAN_POINT('Ctrl Pts',(-52.1027685307223,-17.384247754716,176.951110854015));
#12721=CARTESIAN_POINT('Ctrl Pts',(-51.6569691297711,-17.1812314095055,
177.42208876923));
#12722=CARTESIAN_POINT('Ctrl Pts',(-50.5803007618318,-16.7386138153048,
177.697510231007));
#12723=CARTESIAN_POINT('Ctrl Pts',(-49.9722430688612,-16.5033958825231,
177.495874655633));
#12724=CARTESIAN_POINT('Ctrl Pts',(-49.2598451033921,-16.1323520825764,
176.614580397518));
#12725=CARTESIAN_POINT('Ctrl Pts',(-49.1633964478354,-15.9963838869222,
175.958557394859));
#12726=CARTESIAN_POINT('Ctrl Pts',(-49.6135825845651,-15.8488720097956,
174.863627023648));
#12727=CARTESIAN_POINT('Ctrl Pts',(-50.1513088289339,-15.8357216637453,
174.451396860398));
#12728=CARTESIAN_POINT('Ctrl Pts',(-51.3373123393945,-15.8295083514664,
174.304991255183));
#12729=CARTESIAN_POINT('Ctrl Pts',(-51.9598057434752,-15.8324905082382,
174.577589691682));
#12730=CARTESIAN_POINT('Ctrl Pts',(-52.662356604517,-15.7329936013494,175.540542955831));
#12731=CARTESIAN_POINT('Ctrl Pts',(-52.7287365437827,-15.6278770852026,
176.211335092655));
#12732=CARTESIAN_POINT('Ctrl Pts',(-52.2404503570114,-15.2999892249187,
177.248966419092));
#12733=CARTESIAN_POINT('Ctrl Pts',(-51.7049290320028,-15.079336195701,177.599407337456));
#12734=CARTESIAN_POINT('Ctrl Pts',(-50.599341197491,-14.6318604318474,177.611289749054));
#12735=CARTESIAN_POINT('Ctrl Pts',(-50.0563698831837,-14.4102803084529,
177.271399907022));
#12736=CARTESIAN_POINT('Ctrl Pts',(-49.5511866458666,-14.0779293284932,
176.24060069501));
#12737=CARTESIAN_POINT('Ctrl Pts',(-49.604058679892,-13.971112568136,175.571774049481));
#12738=CARTESIAN_POINT('Ctrl Pts',(-50.2895824050587,-13.8682646399117,
174.596554366676));
#12739=CARTESIAN_POINT('Ctrl Pts',(-50.9089033822508,-13.8698152300494,
174.310925422501));
#12740=CARTESIAN_POINT('Ctrl Pts',(-52.0945937584551,-13.8647732522077,
174.438441317441));
#12741=CARTESIAN_POINT('Ctrl Pts',(-52.6396705452532,-13.8524570813917,
174.840092836798));
#12742=CARTESIAN_POINT('Ctrl Pts',(-53.1114861845869,-13.7091720746061,
175.926135983292));
#12743=CARTESIAN_POINT('Ctrl Pts',(-53.0273981908184,-13.5760746720968,
176.585468457757));
#12744=CARTESIAN_POINT('Ctrl Pts',(-52.3273047331872,-13.2061141571923,
177.480731662196));
#12745=CARTESIAN_POINT('Ctrl Pts',(-51.7260689896615,-12.9732036309654,
177.694033962224));
#12746=CARTESIAN_POINT('Ctrl Pts',(-50.6444965881338,-12.5296009109336,
177.439340266607));
#12747=CARTESIAN_POINT('Ctrl Pts',(-50.1880101288259,-12.323622761024,176.975929902189));
#12748=CARTESIAN_POINT('Ctrl Pts',(-49.9332603826239,-12.0409453485109,
175.846473225312));
#12749=CARTESIAN_POINT('Ctrl Pts',(-50.1325085529845,-11.9618298866148,
175.20357102314));
#12750=CARTESIAN_POINT('Ctrl Pts',(-51.0139495749547,-11.8975707104174,
174.402850839007));
#12751=CARTESIAN_POINT('Ctrl Pts',(-51.6770380739026,-11.9086053392238,
174.263669429449));
#12752=CARTESIAN_POINT('Ctrl Pts',(-52.8102442474793,-11.89211453585,174.644220443453));
#12753=CARTESIAN_POINT('Ctrl Pts',(-53.2534129688289,-11.860550625243,175.158200214442));
#12754=CARTESIAN_POINT('Ctrl Pts',(-53.4727724514858,-11.667970777174,176.317676214963));
#12755=CARTESIAN_POINT('Ctrl Pts',(-53.2447122957938,-11.5059876351892,
176.940267405791));
#12756=CARTESIAN_POINT('Ctrl Pts',(-52.3630606041574,-11.1023742765951,
177.633671542876));
#12757=CARTESIAN_POINT('Ctrl Pts',(-51.7328063873735,-10.863413150139,177.698996091772));
#12758=CARTESIAN_POINT('Ctrl Pts',(-50.7387975664535,-10.4373493069837,
177.194617067458));
#12759=CARTESIAN_POINT('Ctrl Pts',(-50.4003959556136,-10.2552411513015,
176.636362249629));
#12760=CARTESIAN_POINT('Ctrl Pts',(-50.3964887911414,-10.0195709762704,
175.464836254896));
#12761=CARTESIAN_POINT('Ctrl Pts',(-50.7352645697859,-9.96785241001128,
174.878086269107));
#12762=CARTESIAN_POINT('Ctrl Pts',(-51.7761584941716,-9.93363014738946,
174.290073576044));
#12763=CARTESIAN_POINT('Ctrl Pts',(-52.4578743221659,-9.94721824196466,
174.301034748671));
#12764=CARTESIAN_POINT('Ctrl Pts',(-53.4723487166264,-9.90911175935534,
174.927224952557));
#12765=CARTESIAN_POINT('Ctrl Pts',(-53.7905639694071,-9.85304000489839,
175.522456262626));
#12766=CARTESIAN_POINT('Ctrl Pts',(-53.7495974866252,-9.61086987508902,
176.689642787431));
#12767=CARTESIAN_POINT('Ctrl Pts',(-53.3913473444599,-9.42486391207369,
177.234457154129));
#12768=CARTESIAN_POINT('Ctrl Pts',(-52.3804909291071,-8.9950096827268,177.705080880716));
#12769=CARTESIAN_POINT('Ctrl Pts',(-51.7506169575959,-8.75656955580448,
177.617528508224));
#12770=CARTESIAN_POINT('Ctrl Pts',(-50.8938217209944,-8.35631416012115,
176.884644400558));
#12771=CARTESIAN_POINT('Ctrl Pts',(-50.686386739593,-8.19840449522365,176.254364811283));
#12772=CARTESIAN_POINT('Ctrl Pts',(-50.9496816541175,-8.01563271032117,
175.10646784668));
#12773=CARTESIAN_POINT('Ctrl Pts',(-51.4086597834924,-7.98657238824085,
174.608429324338));
#12774=CARTESIAN_POINT('Ctrl Pts',(-52.5506583028891,-7.97253715897243,
174.264721414109));
#12775=CARTESIAN_POINT('Ctrl Pts',(-53.2085070979977,-7.98255305121696,
174.427141629608));
#12776=CARTESIAN_POINT('Ctrl Pts',(-54.0661826067832,-7.91293346685192,
175.257046778597));
#12777=CARTESIAN_POINT('Ctrl Pts',(-54.2443196068901,-7.83026930904402,
175.907383805075));
#12778=CARTESIAN_POINT('Ctrl Pts',(-53.9449265679421,-7.53766373675317,
177.027297077911));
#12779=CARTESIAN_POINT('Ctrl Pts',(-53.4737144264175,-7.32885697968307,
177.474235384447));
#12780=CARTESIAN_POINT('Ctrl Pts',(-52.3866301268079,-6.88556912331281,
177.682767568372));
#12781=CARTESIAN_POINT('Ctrl Pts',(-51.7946034524202,-6.6539762900198,177.44919290535));
#12782=CARTESIAN_POINT('Ctrl Pts',(-51.1242376556131,-6.29031677842802,
176.53135144958));
#12783=CARTESIAN_POINT('Ctrl Pts',(-51.0636455015902,-6.16179111781231,
175.868699032101));
#12784=CARTESIAN_POINT('Ctrl Pts',(-51.5708785507503,-6.02461835391231,
174.795021951807));
#12785=CARTESIAN_POINT('Ctrl Pts',(-52.1305414737447,-6.01557067494389,
174.410384417273));
#12786=CARTESIAN_POINT('Ctrl Pts',(-53.3239707675344,-6.01072022664985,
174.329110015938));
#12787=CARTESIAN_POINT('Ctrl Pts',(-53.9334177584311,-6.01040522494539,
174.634606029695));
#12788=CARTESIAN_POINT('Ctrl Pts',(-54.5783977308191,-5.90111793801205,
175.631553651875));
#12789=CARTESIAN_POINT('Ctrl Pts',(-54.6093650217473,-5.78956533803437,
176.299320421659));
#12790=CARTESIAN_POINT('Ctrl Pts',(-54.0728671794864,-5.45185644429227,
177.309544041851));
#12791=CARTESIAN_POINT('Ctrl Pts',(-53.5182109168208,-5.22801082267814,
177.628618080665));
#12792=CARTESIAN_POINT('Ctrl Pts',(-52.4111095558568,-4.77949537513279,
177.578747218087));
#12793=CARTESIAN_POINT('Ctrl Pts',(-51.8857104064777,-4.56119881916171,
177.207895099161));
#12794=CARTESIAN_POINT('Ctrl Pts',(-51.4375681932236,-4.23993965724606,
176.147216345704));
#12795=CARTESIAN_POINT('Ctrl Pts',(-51.5255341013567,-4.13891120462634,
175.478088476179));
#12796=CARTESIAN_POINT('Ctrl Pts',(-52.2621121714531,-4.04739311840896,
174.545543255356));
#12797=CARTESIAN_POINT('Ctrl Pts',(-52.8911810801,-4.05123090724587,174.294043710706));
#12798=CARTESIAN_POINT('Ctrl Pts',(-54.0705541410016,-4.04422766004653,
174.477498952297));
#12799=CARTESIAN_POINT('Ctrl Pts',(-54.593284417315,-4.02816934534973,174.908686002258));
#12800=CARTESIAN_POINT('Ctrl Pts',(-55.0092587601974,-3.87346271742067,
176.018250487428));
#12801=CARTESIAN_POINT('Ctrl Pts',(-54.8907029615328,-3.73358556412494,
176.67236673678));
#12802=CARTESIAN_POINT('Ctrl Pts',(-54.1422797098421,-3.35431610458726,
177.524634651606));
#12803=CARTESIAN_POINT('Ctrl Pts',(-53.5287781394068,-3.11818277146878,
177.704881014433));
#12804=CARTESIAN_POINT('Ctrl Pts',(-52.4666030700143,-2.67965003658039,
177.385814188219));
#12805=CARTESIAN_POINT('Ctrl Pts',(-52.037952109723,-2.47949238143003,176.900644117435));
#12806=CARTESIAN_POINT('Ctrl Pts',(-51.8369606432704,-2.20643344946428,
175.75693673757));
#12807=CARTESIAN_POINT('Ctrl Pts',(-52.0709636415419,-2.13467360272607,
175.124746251973));
#12808=CARTESIAN_POINT('Ctrl Pts',(-52.9948906247979,-2.07782438513344,
174.368185237747));
#12809=CARTESIAN_POINT('Ctrl Pts',(-53.6658603596095,-2.09023021076396,
174.26394539811));
#12810=CARTESIAN_POINT('Ctrl Pts',(-54.7763899734937,-2.0695796979931,174.705748499134));
#12811=CARTESIAN_POINT('Ctrl Pts',(-55.193636646253,-2.03216929631525,175.243747077929));
#12812=CARTESIAN_POINT('Ctrl Pts',(-55.2990804121262,-1.89289436927212,
176.038719570758));
#12813=CARTESIAN_POINT('Ctrl Pts',(-55.2875271080061,-1.8476232285876,176.255654667139));
#12814=CARTESIAN_POINT('Ctrl Pts',(-55.2062064365128,-1.76817883590891,
176.561034862255));
#12815=CARTESIAN_POINT('Ctrl Pts',(-55.1692797902087,-1.73965218400568,
176.660101738528));
#12816=CARTESIAN_POINT('Ctrl Pts',(-55.100781391479,-1.69439363416682,176.801019080259));
#12817=CARTESIAN_POINT('Ctrl Pts',(-55.0757487692566,-1.67889591755103,
176.846705834293));
#12818=CARTESIAN_POINT('Ctrl Pts',(-55.0215162671022,-1.64716827604208,
176.934897450488));
#12819=CARTESIAN_POINT('Ctrl Pts',(-54.9831012773678,-1.62642361195712,
176.988063802692));
#12820=CARTESIAN_POINT('Ctrl Pts',(-54.9611536226478,-1.61438316700751,
177.018013216499));
#12821=CARTESIAN_POINT('Ctrl Pts',(-49.4509304485228,-27.5317240793367,
176.63793339336));
#12822=CARTESIAN_POINT('Ctrl Pts',(-49.4291393884885,-27.5076562767722,
176.671636728953));
#12823=CARTESIAN_POINT('Ctrl Pts',(-49.4023252814003,-27.49622653535,176.696313164424));
#12824=CARTESIAN_POINT('Ctrl Pts',(-49.3476504462613,-27.4590129437169,
176.750465273433));
#12825=CARTESIAN_POINT('Ctrl Pts',(-49.3184236390985,-27.4399206811032,
176.775937697594));
#12826=CARTESIAN_POINT('Ctrl Pts',(-49.2266057058354,-27.3820561699738,
176.84602259684));
#12827=CARTESIAN_POINT('Ctrl Pts',(-49.1608892759397,-27.3435420466437,
176.883532818161));
#12828=CARTESIAN_POINT('Ctrl Pts',(-48.9520433277106,-27.2233369569446,
176.969216598557));
#12829=CARTESIAN_POINT('Ctrl Pts',(-48.7994772773074,-27.140753695473,176.988359561004));
#12830=CARTESIAN_POINT('Ctrl Pts',(-48.3519200751284,-26.8936813947759,
176.923562975379));
#12831=CARTESIAN_POINT('Ctrl Pts',(-48.0823456895327,-26.734263465041,176.708580257885));
#12832=CARTESIAN_POINT('Ctrl Pts',(-47.8449430900585,-26.4783672905687,
176.126725989992));
#12833=CARTESIAN_POINT('Ctrl Pts',(-47.8767939676907,-26.3778568396964,
175.764012928805));
#12834=CARTESIAN_POINT('Ctrl Pts',(-48.2463197375522,-26.2327937589041,
175.197492946021));
#12835=CARTESIAN_POINT('Ctrl Pts',(-48.5747178643875,-26.1889682126354,
175.01137731386));
#12836=CARTESIAN_POINT('Ctrl Pts',(-49.2462054467177,-26.1087803247027,
174.981703215741));
#12837=CARTESIAN_POINT('Ctrl Pts',(-49.5907543357586,-26.0676212071441,
175.137035562833));
#12838=CARTESIAN_POINT('Ctrl Pts',(-50.009388927793,-25.9343746307825,175.661646016755));
#12839=CARTESIAN_POINT('Ctrl Pts',(-50.0783027352647,-25.8394975457309,
176.025761110018));
#12840=CARTESIAN_POINT('Ctrl Pts',(-49.8988780633176,-25.5959204367964,
176.628597112503));
#12841=CARTESIAN_POINT('Ctrl Pts',(-49.6518990744916,-25.4405710050954,
176.873652740602));
#12842=CARTESIAN_POINT('Ctrl Pts',(-49.0655102948359,-25.1120926941016,
177.024416386827));
#12843=CARTESIAN_POINT('Ctrl Pts',(-48.7382306499136,-24.9412172473198,
176.927283980104));
#12844=CARTESIAN_POINT('Ctrl Pts',(-48.31783324883,-24.6506072191097,176.48408449858));
#12845=CARTESIAN_POINT('Ctrl Pts',(-48.2223197693695,-24.5249427903147,
176.139359044285));
#12846=CARTESIAN_POINT('Ctrl Pts',(-48.3708320195333,-24.3389138358785,
175.495466335841));
#12847=CARTESIAN_POINT('Ctrl Pts',(-48.6129161956615,-24.2782922597527,
175.208867671322));
#12848=CARTESIAN_POINT('Ctrl Pts',(-49.2318343995499,-24.18785243492,174.949625492768));
#12849=CARTESIAN_POINT('Ctrl Pts',(-49.6097264895464,-24.153250081799,174.976039603467));
#12850=CARTESIAN_POINT('Ctrl Pts',(-50.1907740657023,-24.0499499019578,
175.330958269522));
#12851=CARTESIAN_POINT('Ctrl Pts',(-50.3830787723347,-23.9792981329734,
175.653008106489));
#12852=CARTESIAN_POINT('Ctrl Pts',(-50.427159666228,-23.7781136900229,176.297852422263));
#12853=CARTESIAN_POINT('Ctrl Pts',(-50.2832787288339,-23.643180828803,176.621446326487));
#12854=CARTESIAN_POINT('Ctrl Pts',(-49.7924641893585,-23.3338917128074,
176.988303084673));
#12855=CARTESIAN_POINT('Ctrl Pts',(-49.455479895244,-23.1615506277796,177.024112028042));
#12856=CARTESIAN_POINT('Ctrl Pts',(-48.9089639726264,-22.8463871647641,
176.778406765063));
#12857=CARTESIAN_POINT('Ctrl Pts',(-48.699448601228,-22.6985448431478,176.497595410894));
#12858=CARTESIAN_POINT('Ctrl Pts',(-48.6153144001997,-22.4669397150842,
175.854418703293));
#12859=CARTESIAN_POINT('Ctrl Pts',(-48.7438560906085,-22.3839338201049,
175.504557803726));
#12860=CARTESIAN_POINT('Ctrl Pts',(-49.2595227997445,-22.2634194140522,
175.031489327737));
#12861=CARTESIAN_POINT('Ctrl Pts',(-49.6731287428438,-22.2242903845664,
174.93387435438));
#12862=CARTESIAN_POINT('Ctrl Pts',(-50.3871280758708,-22.1273049999089,
175.149675576275));
#12863=CARTESIAN_POINT('Ctrl Pts',(-50.6724659987737,-22.0667095289654,
175.454257853488));
#12864=CARTESIAN_POINT('Ctrl Pts',(-50.8432291330538,-21.8630647724227,
176.162580877915));
#12865=CARTESIAN_POINT('Ctrl Pts',(-50.7223573298116,-21.7238000115757,
176.543315008655));
#12866=CARTESIAN_POINT('Ctrl Pts',(-50.2109398093855,-21.3899066275767,
176.985840165295));
#12867=CARTESIAN_POINT('Ctrl Pts',(-49.8297406934723,-21.1967740899633,
177.034608068765));
#12868=CARTESIAN_POINT('Ctrl Pts',(-49.2383022679982,-20.8522162432738,
176.742643808163));
#12869=CARTESIAN_POINT('Ctrl Pts',(-49.0288695410029,-20.692930608689,176.406589078903));
#12870=CARTESIAN_POINT('Ctrl Pts',(-49.026421127215,-20.4577766282769,175.692082743004));
#12871=CARTESIAN_POINT('Ctrl Pts',(-49.2307435857662,-20.3815547180372,
175.331094438645));
#12872=CARTESIAN_POINT('Ctrl Pts',(-49.8766835352141,-20.269544445424,174.953525304613));
#12873=CARTESIAN_POINT('Ctrl Pts',(-50.2982947167721,-20.234888952096,174.950394529643));
#12874=CARTESIAN_POINT('Ctrl Pts',(-50.9484787003876,-20.125016744292,175.316388781725));
#12875=CARTESIAN_POINT('Ctrl Pts',(-51.1618775184403,-20.046547250015,175.681463428659));
#12876=CARTESIAN_POINT('Ctrl Pts',(-51.1680956128,-19.8172503157992,176.389348367045));
#12877=CARTESIAN_POINT('Ctrl Pts',(-50.9669054157941,-19.6595598406301,
176.731136037536));
#12878=CARTESIAN_POINT('Ctrl Pts',(-50.3735191706099,-19.3104097045359,
177.03446439702));
#12879=CARTESIAN_POINT('Ctrl Pts',(-49.9983681415115,-19.122445314997,176.992069263085));
#12880=CARTESIAN_POINT('Ctrl Pts',(-49.4783291859613,-18.7856098039383,
176.558083132201));
#12881=CARTESIAN_POINT('Ctrl Pts',(-49.3516920035876,-18.6452157185327,
176.179591346513));
#12882=CARTESIAN_POINT('Ctrl Pts',(-49.5099669630901,-18.4404938180664,
175.471248155379));
#12883=CARTESIAN_POINT('Ctrl Pts',(-49.7966826107081,-18.3761869903911,
175.157298861455));
#12884=CARTESIAN_POINT('Ctrl Pts',(-50.5005002255267,-18.2813908051205,
174.934848239897));
#12885=CARTESIAN_POINT('Ctrl Pts',(-50.9163195448478,-18.2427172185017,
175.022527695559));
#12886=CARTESIAN_POINT('Ctrl Pts',(-51.4689900750814,-18.1145211614547,
175.516882458909));
#12887=CARTESIAN_POINT('Ctrl Pts',(-51.5957313663424,-18.0233261232984,
175.908710828391));
#12888=CARTESIAN_POINT('Ctrl Pts',(-51.4475718943418,-17.7582443007608,
176.601404917962));
#12889=CARTESIAN_POINT('Ctrl Pts',(-51.1767645681398,-17.5900571721881,
176.879541091562));
#12890=CARTESIAN_POINT('Ctrl Pts',(-50.5307383316194,-17.2301836239675,
177.028185493998));
#12891=CARTESIAN_POINT('Ctrl Pts',(-50.1698955770676,-17.0410908031352,
176.891376748831));
#12892=CARTESIAN_POINT('Ctrl Pts',(-49.7689671613288,-16.733171977968,176.344861065041));
#12893=CARTESIAN_POINT('Ctrl Pts',(-49.7283236820348,-16.606509721343,175.939499115166));
#12894=CARTESIAN_POINT('Ctrl Pts',(-50.039329025483,-16.4317046321664,175.276913396961));
#12895=CARTESIAN_POINT('Ctrl Pts',(-50.3811663065111,-16.3819545297351,
175.034692629757));
#12896=CARTESIAN_POINT('Ctrl Pts',(-51.1285550225506,-16.289595439286,174.965429755586));
#12897=CARTESIAN_POINT('Ctrl Pts',(-51.5107791504261,-16.247329788901,175.141829956289));
#12898=CARTESIAN_POINT('Ctrl Pts',(-51.9410271179475,-16.0950193648309,
175.742297045045));
#12899=CARTESIAN_POINT('Ctrl Pts',(-51.9772772372669,-15.9825461483302,
176.155328152494));
#12900=CARTESIAN_POINT('Ctrl Pts',(-51.6813604170028,-15.6948169276305,
176.775145838897));
#12901=CARTESIAN_POINT('Ctrl Pts',(-51.3553093740791,-15.5131006527082,
176.981869312707));
#12902=CARTESIAN_POINT('Ctrl Pts',(-50.6958293220101,-15.1512003838696,
176.968860943967));
#12903=CARTESIAN_POINT('Ctrl Pts',(-50.3793004471536,-14.974461104635,176.752883253889));
#12904=CARTESIAN_POINT('Ctrl Pts',(-50.1044053585231,-14.6849545931669,
176.110550614429));
#12905=CARTESIAN_POINT('Ctrl Pts',(-50.1562892256051,-14.5790344049375,
175.704381183727));
#12906=CARTESIAN_POINT('Ctrl Pts',(-50.6091148636379,-14.4310075872896,
175.119365593043));
#12907=CARTESIAN_POINT('Ctrl Pts',(-51.0040002342342,-14.3877335732316,
174.956144468714));
#12908=CARTESIAN_POINT('Ctrl Pts',(-51.7368765161625,-14.2984333198446,
175.052400920313));
#12909=CARTESIAN_POINT('Ctrl Pts',(-52.0746787278137,-14.2446881736679,
175.307721150405));
#12910=CARTESIAN_POINT('Ctrl Pts',(-52.3618029222314,-14.0653384618121,
175.979593696432));
#12911=CARTESIAN_POINT('Ctrl Pts',(-52.3085224478133,-13.9393545956389,
176.378830696363));
#12912=CARTESIAN_POINT('Ctrl Pts',(-51.8806097785072,-13.6203167705008,
176.914733769747));
#12913=CARTESIAN_POINT('Ctrl Pts',(-51.5196766160896,-13.4348339691437,
177.033422941425));
#12914=CARTESIAN_POINT('Ctrl Pts',(-50.8796650354229,-13.0760747213028,
176.857816848924));
#12915=CARTESIAN_POINT('Ctrl Pts',(-50.6171262914928,-12.905954023484,176.563294278628));
#12916=CARTESIAN_POINT('Ctrl Pts',(-50.4974416512911,-12.6523824704848,
175.874038771655));
#12917=CARTESIAN_POINT('Ctrl Pts',(-50.6384867622314,-12.5605842376971,
175.481424733232));
#12918=CARTESIAN_POINT('Ctrl Pts',(-51.2082627201524,-12.4357774521296,
175.006422958104));
#12919=CARTESIAN_POINT('Ctrl Pts',(-51.6220204445227,-12.3999030775176,
174.932310130414));
#12920=CARTESIAN_POINT('Ctrl Pts',(-52.3278760969134,-12.2994377602634,
175.185413156184));
#12921=CARTESIAN_POINT('Ctrl Pts',(-52.5969267492371,-12.2353856775628,
175.505423112887));
#12922=CARTESIAN_POINT('Ctrl Pts',(-52.7283564524999,-12.0255423744405,
176.2175433277));
#12923=CARTESIAN_POINT('Ctrl Pts',(-52.5846730379872,-11.8782873041682,
176.594912064781));
#12924=CARTESIAN_POINT('Ctrl Pts',(-52.0559417647627,-11.5457913524836,
176.999632681105));
#12925=CARTESIAN_POINT('Ctrl Pts',(-51.6759748702359,-11.3536364027873,
177.029489895259));
#12926=CARTESIAN_POINT('Ctrl Pts',(-51.0935427887116,-11.0064931497742,
176.702663500826));
#12927=CARTESIAN_POINT('Ctrl Pts',(-50.9048767955961,-10.8544314216914,
176.357244031546));
#12928=CARTESIAN_POINT('Ctrl Pts',(-50.9399834898308,-10.6247204655602,
175.63759182164));
#12929=CARTESIAN_POINT('Ctrl Pts',(-51.1643267174014,-10.5520247194105,
175.286394351447));
#12930=CARTESIAN_POINT('Ctrl Pts',(-51.827873009513,-10.4447251212865,174.944424130566));
#12931=CARTESIAN_POINT('Ctrl Pts',(-52.2552179028772,-10.4077182802165,
174.964702471846));
#12932=CARTESIAN_POINT('Ctrl Pts',(-52.8763669051787,-10.2968258721765,
175.360239151239));
#12933=CARTESIAN_POINT('Ctrl Pts',(-53.071683414474,-10.215593033151,175.73103698433));
#12934=CARTESIAN_POINT('Ctrl Pts',(-53.0437675059112,-9.97549498249197,
176.443487491333));
#12935=CARTESIAN_POINT('Ctrl Pts',(-52.825568431635,-9.81766629245078,176.768582048511));
#12936=CARTESIAN_POINT('Ctrl Pts',(-52.2143534856381,-9.46331409552581,
177.038351228206));
#12937=CARTESIAN_POINT('Ctrl Pts',(-51.8411412849432,-9.27545967967225,
176.973585868646));
#12938=CARTESIAN_POINT('Ctrl Pts',(-51.3467118649778,-8.94477024831946,
176.509526159241));
#12939=CARTESIAN_POINT('Ctrl Pts',(-51.2404836863797,-8.80483732687828,
176.117599105019));
#12940=CARTESIAN_POINT('Ctrl Pts',(-51.4349583516297,-8.61185430488912,
175.425788146171));
#12941=CARTESIAN_POINT('Ctrl Pts',(-51.7335486000159,-8.55040314694308,
175.126384517701));
#12942=CARTESIAN_POINT('Ctrl Pts',(-52.4549196826756,-8.45481293341497,
174.935526629257));
#12943=CARTESIAN_POINT('Ctrl Pts',(-52.8607223331575,-8.41739346719437,
175.04474867484));
#12944=CARTESIAN_POINT('Ctrl Pts',(-53.3897252776085,-8.28282809274167,
175.568595073035));
#12945=CARTESIAN_POINT('Ctrl Pts',(-53.4952826969923,-8.1872595086965,175.966830212787));
#12946=CARTESIAN_POINT('Ctrl Pts',(-53.3101642867802,-7.91637813164073,
176.645610777581));
#12947=CARTESIAN_POINT('Ctrl Pts',(-53.02056762136,-7.74105352934409,176.910070201754));
#12948=CARTESIAN_POINT('Ctrl Pts',(-52.3751524190461,-7.38599804306437,
177.017607675131));
#12949=CARTESIAN_POINT('Ctrl Pts',(-52.0232566558232,-7.19924964083975,
176.864225220861));
#12950=CARTESIAN_POINT('Ctrl Pts',(-51.6458284953554,-6.89163712519652,
176.29020971736));
#12951=CARTESIAN_POINT('Ctrl Pts',(-51.6277644578821,-6.7724816775637,175.885858382765));
#12952=CARTESIAN_POINT('Ctrl Pts',(-51.9747906942483,-6.6028499237395,175.235443151034));
#12953=CARTESIAN_POINT('Ctrl Pts',(-52.3299962525585,-6.55546850196264,
175.011060208135));
#12954=CARTESIAN_POINT('Ctrl Pts',(-53.0782096175287,-6.46444741567071,
174.9816560919));
#12955=CARTESIAN_POINT('Ctrl Pts',(-53.4553178435249,-6.41778988524295,
175.181401713961));
#12956=CARTESIAN_POINT('Ctrl Pts',(-53.8466529433518,-6.26265155715774,
175.795420851333));
#12957=CARTESIAN_POINT('Ctrl Pts',(-53.864188958285,-6.14704492720176,176.206287912404));
#12958=CARTESIAN_POINT('Ctrl Pts',(-53.5358416511927,-5.84903598495515,
176.813977641948));
#12959=CARTESIAN_POINT('Ctrl Pts',(-53.2017653978813,-5.66889429660941,
176.99856451113));
#12960=CARTESIAN_POINT('Ctrl Pts',(-52.5405403606902,-5.30479587533914,
176.947248559284));
#12961=CARTESIAN_POINT('Ctrl Pts',(-52.2356929075399,-5.13012364220884,
176.712058308829));
#12962=CARTESIAN_POINT('Ctrl Pts',(-51.9967219623743,-4.84888631606004,
176.054758979681));
#12963=CARTESIAN_POINT('Ctrl Pts',(-52.0727509238964,-4.74401755802611,
175.645031481929));
#12964=CARTESIAN_POINT('Ctrl Pts',(-52.5505176724514,-4.6056507589775,175.091566392661));
#12965=CARTESIAN_POINT('Ctrl Pts',(-52.9499574883172,-4.56374410570602,
174.946492448473));
#12966=CARTESIAN_POINT('Ctrl Pts',(-53.685231908784,-4.47066113931358,175.078743542747));
#12967=CARTESIAN_POINT('Ctrl Pts',(-54.0046084640979,-4.41655583760205,
175.349203817777));
#12968=CARTESIAN_POINT('Ctrl Pts',(-54.2577428662421,-4.2288827567675,176.036685454146));
#12969=CARTESIAN_POINT('Ctrl Pts',(-54.1828214302285,-4.09851492101137,
176.431966849275));
#12970=CARTESIAN_POINT('Ctrl Pts',(-53.7276699197103,-3.77548143923658,
176.939160233154));
#12971=CARTESIAN_POINT('Ctrl Pts',(-53.3559275609679,-3.58443131799679,
177.036850521868));
#12972=CARTESIAN_POINT('Ctrl Pts',(-52.7340684542075,-3.23387064793483,
176.825149499914));
#12973=CARTESIAN_POINT('Ctrl Pts',(-52.4865052787647,-3.06716804391598,
176.519600526728));
#12974=CARTESIAN_POINT('Ctrl Pts',(-52.4000162427049,-2.81575249291398,
175.815720536334));
#12975=CARTESIAN_POINT('Ctrl Pts',(-52.5606356723736,-2.73100846880393,
175.434725535823));
#12976=CARTESIAN_POINT('Ctrl Pts',(-53.1578253291134,-2.60958353788362,
174.986380686329));
#12977=CARTESIAN_POINT('Ctrl Pts',(-53.575919582614,-2.57427864177586,174.934476257966));
#12978=CARTESIAN_POINT('Ctrl Pts',(-54.2645385526377,-2.47204238084449,
175.223470220004));
#12979=CARTESIAN_POINT('Ctrl Pts',(-54.5189943505689,-2.4021627120238,175.561903562137));
#12980=CARTESIAN_POINT('Ctrl Pts',(-54.5814297773468,-2.25612793931688,
176.045419377677));
#12981=CARTESIAN_POINT('Ctrl Pts',(-54.5735173041519,-2.21013144506474,
176.178993521001));
#12982=CARTESIAN_POINT('Ctrl Pts',(-54.5239654997844,-2.13806319233694,
176.36226950621));
#12983=CARTESIAN_POINT('Ctrl Pts',(-54.5010361022764,-2.1121733501921,176.42270110964));
#12984=CARTESIAN_POINT('Ctrl Pts',(-54.4586925003588,-2.07172971741335,
176.508171829538));
#12985=CARTESIAN_POINT('Ctrl Pts',(-54.4432559654462,-2.05799768545568,
176.53580222906));
#12986=CARTESIAN_POINT('Ctrl Pts',(-54.410122331684,-2.03029642349882,176.588723178982));
#12987=CARTESIAN_POINT('Ctrl Pts',(-54.3884821434676,-2.0139079395113,176.618668306411));
#12988=CARTESIAN_POINT('Ctrl Pts',(-54.3738267566562,-2.00237092626598,
176.637865020199));
#12989=CARTESIAN_POINT('Ctrl Pts',(-49.6057233026533,-28.1882175989763,
177.068114089093));
#12990=CARTESIAN_POINT('Ctrl Pts',(-49.5663192275732,-28.1656109096198,
177.105925367078));
#12991=CARTESIAN_POINT('Ctrl Pts',(-49.5216854287654,-28.1457023853521,
177.148383027181));
#12992=CARTESIAN_POINT('Ctrl Pts',(-49.4301127133764,-28.1014695235449,
177.220446553382));
#12993=CARTESIAN_POINT('Ctrl Pts',(-49.3819809603125,-28.0788363277035,
177.253617740645));
#12994=CARTESIAN_POINT('Ctrl Pts',(-49.2321484222821,-28.0099337266433,
177.343479018307));
#12995=CARTESIAN_POINT('Ctrl Pts',(-49.1254026293825,-27.9629901656525,
177.390284377819));
#12996=CARTESIAN_POINT('Ctrl Pts',(-48.7929164986652,-27.8189908160803,
177.48590296908));
#12997=CARTESIAN_POINT('Ctrl Pts',(-48.55635218661,-27.7202377019268,177.490394220553));
#12998=CARTESIAN_POINT('Ctrl Pts',(-47.8840648999533,-27.4305281812212,
177.324447440169));
#12999=CARTESIAN_POINT('Ctrl Pts',(-47.5006474873523,-27.2497443022818,
176.963331771584));
#13000=CARTESIAN_POINT('Ctrl Pts',(-47.2040861213115,-26.9802047380462,
176.046394548579));
#13001=CARTESIAN_POINT('Ctrl Pts',(-47.2954018922066,-26.8917044501032,
175.506598760119));
#13002=CARTESIAN_POINT('Ctrl Pts',(-47.9062028356891,-26.7943163650827,
174.710326627486));
#13003=CARTESIAN_POINT('Ctrl Pts',(-48.4108882632775,-26.7850298620733,
174.47568647468));
#13004=CARTESIAN_POINT('Ctrl Pts',(-49.4081207961382,-26.7654318876047,
174.522051214009));
#13005=CARTESIAN_POINT('Ctrl Pts',(-49.8895805322777,-26.7512165827191,
174.803706734764));
#13006=CARTESIAN_POINT('Ctrl Pts',(-50.419859907048,-26.6406327974915,175.641132157405));
#13007=CARTESIAN_POINT('Ctrl Pts',(-50.4638072135826,-26.5414518590087,
176.190943138814));
#13008=CARTESIAN_POINT('Ctrl Pts',(-50.0902675056585,-26.258306693899,177.06820282525));
#13009=CARTESIAN_POINT('Ctrl Pts',(-49.6753169680471,-26.0710530131776,
177.393289133135));
#13010=CARTESIAN_POINT('Ctrl Pts',(-48.760110273011,-25.6803067135432,177.526354227003));
#13011=CARTESIAN_POINT('Ctrl Pts',(-48.2752065557733,-25.4795815288234,
177.333261554155));
#13012=CARTESIAN_POINT('Ctrl Pts',(-47.6834949732814,-25.1537104488559,
176.598820399841));
#13013=CARTESIAN_POINT('Ctrl Pts',(-47.581935800625,-25.0274199406948,176.066471856633));
#13014=CARTESIAN_POINT('Ctrl Pts',(-47.8743577335121,-24.8702793490883,
175.122570330099));
#13015=CARTESIAN_POINT('Ctrl Pts',(-48.2639300332364,-24.8386062285325,
174.72605490093));
#13016=CARTESIAN_POINT('Ctrl Pts',(-49.2134664973944,-24.8097944361078,
174.418869413643));
#13017=CARTESIAN_POINT('Ctrl Pts',(-49.7639560285487,-24.8089577046691,
174.513086690221));
#13018=CARTESIAN_POINT('Ctrl Pts',(-50.5601436025432,-24.7482854574026,
175.121296078095));
#13019=CARTESIAN_POINT('Ctrl Pts',(-50.7937850628585,-24.6861522884041,
175.625415363842));
#13020=CARTESIAN_POINT('Ctrl Pts',(-50.7513118113109,-24.4660502953853,
176.598470930813));
#13021=CARTESIAN_POINT('Ctrl Pts',(-50.4787452748198,-24.3068424850894,
177.056448064075));
#13022=CARTESIAN_POINT('Ctrl Pts',(-49.6755858463959,-23.9384579984121,
177.525629368769));
#13023=CARTESIAN_POINT('Ctrl Pts',(-49.1583261106009,-23.7318611386462,
177.529378707235));
#13024=CARTESIAN_POINT('Ctrl Pts',(-48.3492917504345,-23.3639427741862,
177.074636497803));
#13025=CARTESIAN_POINT('Ctrl Pts',(-48.0678997211374,-23.2027238239874,
176.620161976926));
#13026=CARTESIAN_POINT('Ctrl Pts',(-48.0133698591323,-22.9779683240005,
175.643265853549));
#13027=CARTESIAN_POINT('Ctrl Pts',(-48.2419634078688,-22.9148026311583,
175.13669620061));
#13028=CARTESIAN_POINT('Ctrl Pts',(-49.0648716087653,-22.8512007031896,
174.491772947554));
#13029=CARTESIAN_POINT('Ctrl Pts',(-49.6839608902416,-22.8528771386521,
174.405900021421));
#13030=CARTESIAN_POINT('Ctrl Pts',(-50.6991943315865,-22.8143164724711,
174.826217042058));
#13031=CARTESIAN_POINT('Ctrl Pts',(-51.0745700439279,-22.7701586995258,
175.322569579276));
#13032=CARTESIAN_POINT('Ctrl Pts',(-51.2073695092728,-22.5604456438022,
176.396956445951));
#13033=CARTESIAN_POINT('Ctrl Pts',(-50.9625278765238,-22.3963905325425,
176.94851178212));
#13034=CARTESIAN_POINT('Ctrl Pts',(-50.1139689940341,-21.9977514714476,
177.529315681618));
#13035=CARTESIAN_POINT('Ctrl Pts',(-49.5293219694751,-21.7666067892758,
177.544699935169));
#13036=CARTESIAN_POINT('Ctrl Pts',(-48.6567664449969,-21.3653910132907,
177.013098304479));
#13037=CARTESIAN_POINT('Ctrl Pts',(-48.383128531039,-21.1949054338945,176.477577858981));
#13038=CARTESIAN_POINT('Ctrl Pts',(-48.4582777380059,-20.975048733324,175.402873064259));
#13039=CARTESIAN_POINT('Ctrl Pts',(-48.8055781932514,-20.9254744005303,
174.886960050279));
#13040=CARTESIAN_POINT('Ctrl Pts',(-49.7998797569528,-20.8818943796597,
174.412232108109));
#13041=CARTESIAN_POINT('Ctrl Pts',(-50.4230224397188,-20.885216808613,174.464849386198));
#13042=CARTESIAN_POINT('Ctrl Pts',(-51.3220781362712,-20.8236066704411,
175.100442044691));
#13043=CARTESIAN_POINT('Ctrl Pts',(-51.5785314568021,-20.7546592125729,
175.670463366294));
#13044=CARTESIAN_POINT('Ctrl Pts',(-51.4682882413066,-20.5004564781585,
176.732562819156));
#13045=CARTESIAN_POINT('Ctrl Pts',(-51.1076577914431,-20.313201754554,177.207532153307));
#13046=CARTESIAN_POINT('Ctrl Pts',(-50.156411198824,-19.8953744930702,177.56803029022));
#13047=CARTESIAN_POINT('Ctrl Pts',(-49.5878400685962,-19.6691878319784,
177.446385146947));
#13048=CARTESIAN_POINT('Ctrl Pts',(-48.852079415717,-19.2920053425884,176.716949064536));
#13049=CARTESIAN_POINT('Ctrl Pts',(-48.7034574890464,-19.1464856081966,
176.127114392609));
#13050=CARTESIAN_POINT('Ctrl Pts',(-49.017896392823,-18.9721498737463,175.084671234462));
#13051=CARTESIAN_POINT('Ctrl Pts',(-49.4761175027563,-18.9421345006494,
174.655217811997));
#13052=CARTESIAN_POINT('Ctrl Pts',(-50.5469446991098,-18.915664221674,174.415005106013));
#13053=CARTESIAN_POINT('Ctrl Pts',(-51.1421889783774,-18.9127734302845,
174.605352538579));
#13054=CARTESIAN_POINT('Ctrl Pts',(-51.8771202801842,-18.8200557591642,
175.418505113175));
#13055=CARTESIAN_POINT('Ctrl Pts',(-52.0018165496213,-18.7275436462981,
176.022835099282));
#13056=CARTESIAN_POINT('Ctrl Pts',(-51.6614363875286,-18.4266465795959,
177.027259608014));
#13057=CARTESIAN_POINT('Ctrl Pts',(-51.2055166082591,-18.2218754080822,
177.403206831321));
#13058=CARTESIAN_POINT('Ctrl Pts',(-50.1969770591628,-17.7923688711786,
177.524973109627));
#13059=CARTESIAN_POINT('Ctrl Pts',(-49.6679526067506,-17.5720619524455,
177.267256975221));
#13060=CARTESIAN_POINT('Ctrl Pts',(-49.1179984398299,-17.2329564925234,
176.379271882249));
#13061=CARTESIAN_POINT('Ctrl Pts',(-49.1058293111544,-17.1129691055462,
175.766207634738));
#13062=CARTESIAN_POINT('Ctrl Pts',(-49.6421979468107,-16.981953011196,174.814805282058));
#13063=CARTESIAN_POINT('Ctrl Pts',(-50.1794692968359,-16.96896833752,174.497498655776));
#13064=CARTESIAN_POINT('Ctrl Pts',(-51.2815033366288,-16.9462509137644,
174.497183387712));
#13065=CARTESIAN_POINT('Ctrl Pts',(-51.8206810039433,-16.9333636766774,
174.813868002799));
#13066=CARTESIAN_POINT('Ctrl Pts',(-52.3579329121243,-16.8019633847227,
175.767995550527));
#13067=CARTESIAN_POINT('Ctrl Pts',(-52.3444015552563,-16.6811074119364,
176.384253300385));
#13068=CARTESIAN_POINT('Ctrl Pts',(-51.7908025496479,-16.3412377353734,
177.270036214878));
#13069=CARTESIAN_POINT('Ctrl Pts',(-51.2640575414935,-16.1220052064028,
177.524939199898));
#13070=CARTESIAN_POINT('Ctrl Pts',(-50.2584821099884,-15.6936926334193,
177.402964762685));
#13071=CARTESIAN_POINT('Ctrl Pts',(-49.8024659570259,-15.4891340123335,
177.028965203342));
#13072=CARTESIAN_POINT('Ctrl Pts',(-49.4615190985809,-15.1881425443655,
176.024838210267));
#13073=CARTESIAN_POINT('Ctrl Pts',(-49.584917871472,-15.0951235636284,175.418993178211));
#13074=CARTESIAN_POINT('Ctrl Pts',(-50.3224323861862,-15.0022736039987,
174.603877612758));
#13075=CARTESIAN_POINT('Ctrl Pts',(-50.9209588419739,-14.9994851008446,
174.413907495741));
#13076=CARTESIAN_POINT('Ctrl Pts',(-51.9913299824675,-14.9728180278691,
174.658436700836));
#13077=CARTESIAN_POINT('Ctrl Pts',(-52.4458562262816,-14.942768055369,175.086526075902));
#13078=CARTESIAN_POINT('Ctrl Pts',(-52.7589234637054,-14.768747576336,176.126312497655));
#13079=CARTESIAN_POINT('Ctrl Pts',(-52.6119738826496,-14.6237809758753,
176.715478760326));
#13080=CARTESIAN_POINT('Ctrl Pts',(-51.8767097042875,-14.2467264136774,
177.445252299972));
#13081=CARTESIAN_POINT('Ctrl Pts',(-51.3074205647036,-14.0201741438431,
177.568755188896));
#13082=CARTESIAN_POINT('Ctrl Pts',(-50.3534291722187,-13.6011459302421,
177.20657523661));
#13083=CARTESIAN_POINT('Ctrl Pts',(-49.9921349812078,-13.4131957453291,
176.728222347554));
#13084=CARTESIAN_POINT('Ctrl Pts',(-49.8860852889645,-13.159806046502,175.66552302478));
#13085=CARTESIAN_POINT('Ctrl Pts',(-50.1425376823364,-13.0914495220188,
175.099033652958));
#13086=CARTESIAN_POINT('Ctrl Pts',(-51.0393482876635,-13.0300320803285,
174.465742160163));
#13087=CARTESIAN_POINT('Ctrl Pts',(-51.661049564308,-13.0333384108268,174.411629490546));
#13088=CARTESIAN_POINT('Ctrl Pts',(-52.6556849728402,-12.9898139344045,
174.885756683857));
#13089=CARTESIAN_POINT('Ctrl Pts',(-53.0050117718212,-12.9403514819039,
175.401975295897));
#13090=CARTESIAN_POINT('Ctrl Pts',(-53.0797917942593,-12.7198628954119,
176.47950485369));
#13091=CARTESIAN_POINT('Ctrl Pts',(-52.8035180796908,-12.5482535501767,
177.017249165378));
#13092=CARTESIAN_POINT('Ctrl Pts',(-51.928756778869,-12.1465816152287,177.545168184464));
#13093=CARTESIAN_POINT('Ctrl Pts',(-51.3476399628683,-11.9168238447545,
177.52855345072));
#13094=CARTESIAN_POINT('Ctrl Pts',(-50.5013329357435,-11.5191203268418,
176.948730973903));
#13095=CARTESIAN_POINT('Ctrl Pts',(-50.2557375091139,-11.3551615877155,
176.398843509589));
#13096=CARTESIAN_POINT('Ctrl Pts',(-50.3877927376681,-11.145398461788,175.324825412843));
#13097=CARTESIAN_POINT('Ctrl Pts',(-50.762684868614,-11.1008426423184,174.826271833705));
#13098=CARTESIAN_POINT('Ctrl Pts',(-51.7811268292925,-11.0622619854364,
174.405264562934));
#13099=CARTESIAN_POINT('Ctrl Pts',(-52.4028793467296,-11.063958202758,174.492793292778));
#13100=CARTESIAN_POINT('Ctrl Pts',(-53.2632154661256,-10.9967409315864,
175.172494096186));
#13101=CARTESIAN_POINT('Ctrl Pts',(-53.4886849878534,-10.9225114509841,
175.750866168407));
#13102=CARTESIAN_POINT('Ctrl Pts',(-53.3251423960266,-10.6565821386363,
176.805379202472));
#13103=CARTESIAN_POINT('Ctrl Pts',(-52.9407422532226,-10.465785944074,177.259010843821));
#13104=CARTESIAN_POINT('Ctrl Pts',(-51.9697953271392,-10.0433159226031,
177.565260787091));
#13105=CARTESIAN_POINT('Ctrl Pts',(-51.4073968434514,-9.81808614025534,
177.411394538556));
#13106=CARTESIAN_POINT('Ctrl Pts',(-50.7116066211125,-9.44884954788431,
176.639139203566));
#13107=CARTESIAN_POINT('Ctrl Pts',(-50.5960828064805,-9.30833579234248,
176.038056438509));
#13108=CARTESIAN_POINT('Ctrl Pts',(-50.9640903737478,-9.14636922546571,
175.0167568496));
#13109=CARTESIAN_POINT('Ctrl Pts',(-51.4414488535671,-9.12058052193367,
174.612974652851));
#13110=CARTESIAN_POINT('Ctrl Pts',(-52.5249204417031,-9.09513784416194,
174.426509843431));
#13111=CARTESIAN_POINT('Ctrl Pts',(-53.1088418277628,-9.09114996369398,
174.646804488947));
#13112=CARTESIAN_POINT('Ctrl Pts',(-53.801661971168,-8.98942785386125,175.498626413927));
#13113=CARTESIAN_POINT('Ctrl Pts',(-53.8945655335682,-8.89052591977855,
176.108945227942));
#13114=CARTESIAN_POINT('Ctrl Pts',(-53.5007325042087,-8.57967938234873,
177.090495387502));
#13115=CARTESIAN_POINT('Ctrl Pts',(-53.0228734977247,-8.36926263084827,
177.439659990072));
#13116=CARTESIAN_POINT('Ctrl Pts',(-52.0134388460396,-7.941561484533,177.502665384752));
#13117=CARTESIAN_POINT('Ctrl Pts',(-51.5009539686643,-7.72503451842822,
177.217498325365));
#13118=CARTESIAN_POINT('Ctrl Pts',(-50.9958226444158,-7.39311721565184,
176.298072843289));
#13119=CARTESIAN_POINT('Ctrl Pts',(-51.0149583411939,-7.28021855779389,
175.684524900703));
#13120=CARTESIAN_POINT('Ctrl Pts',(-51.602189663565,-7.15816051285745,174.759352960774));
#13121=CARTESIAN_POINT('Ctrl Pts',(-52.1561751142271,-7.14821693453925,
174.470064567704));
#13122=CARTESIAN_POINT('Ctrl Pts',(-53.257284967077,-7.12553378294388,174.528734890764));
#13123=CARTESIAN_POINT('Ctrl Pts',(-53.7798318899166,-7.10813319884164,
174.876062446534));
#13124=CARTESIAN_POINT('Ctrl Pts',(-54.263309402104,-6.96831483361839,175.852098283111));
#13125=CARTESIAN_POINT('Ctrl Pts',(-54.2182177005742,-6.84182185515181,
176.463118413));
#13126=CARTESIAN_POINT('Ctrl Pts',(-53.620326169719,-6.49215310837908,177.317242942806));
#13127=CARTESIAN_POINT('Ctrl Pts',(-53.0815432796407,-6.27162057701451,
177.542753252723));
#13128=CARTESIAN_POINT('Ctrl Pts',(-52.0813405764902,-5.84340716815714,
177.363069610828));
#13129=CARTESIAN_POINT('Ctrl Pts',(-51.6451899827477,-5.64252013198273,
176.962963727015));
#13130=CARTESIAN_POINT('Ctrl Pts',(-51.3585173428123,-5.35236886702559,
175.939011043839));
#13131=CARTESIAN_POINT('Ctrl Pts',(-51.5164782073777,-5.2645103327986,175.337256223397));
#13132=CARTESIAN_POINT('Ctrl Pts',(-52.2924300679745,-5.18119763163266,
174.565366155634));
#13133=CARTESIAN_POINT('Ctrl Pts',(-52.8973452213176,-5.1801045826173,174.406680096152));
#13134=CARTESIAN_POINT('Ctrl Pts',(-53.956162505713,-5.14973256956073,174.705214074754));
#13135=CARTESIAN_POINT('Ctrl Pts',(-54.3874707400874,-5.11629663400306,
175.155234787811));
#13136=CARTESIAN_POINT('Ctrl Pts',(-54.6460006492434,-4.93091655090319,
176.210608238885));
#13137=CARTESIAN_POINT('Ctrl Pts',(-54.4681690759566,-4.77980797892323,
176.790635503925));
#13138=CARTESIAN_POINT('Ctrl Pts',(-53.6946945331643,-4.3956772156615,177.47627897342));
#13139=CARTESIAN_POINT('Ctrl Pts',(-53.1174419759953,-4.16620647621949,
177.565792133827));
#13140=CARTESIAN_POINT('Ctrl Pts',(-52.1878574222778,-3.75385530866336,
177.150829002666));
#13141=CARTESIAN_POINT('Ctrl Pts',(-51.8529856411974,-3.5715083216093,176.654958973924));
#13142=CARTESIAN_POINT('Ctrl Pts',(-51.8010050251376,-3.32706416715232,
175.583828138226));
#13143=CARTESIAN_POINT('Ctrl Pts',(-52.0854219579878,-3.26527816982496,
175.031488604324));
#13144=CARTESIAN_POINT('Ctrl Pts',(-53.0170398348192,-3.20959915076688,
174.444132662069));
#13145=CARTESIAN_POINT('Ctrl Pts',(-53.6416591927321,-3.21325709639781,
174.423035709656));
#13146=CARTESIAN_POINT('Ctrl Pts',(-54.6090153740635,-3.16498595686182,
174.948967905512));
#13147=CARTESIAN_POINT('Ctrl Pts',(-54.9308286711417,-3.10893139642228,
175.48555871107));
#13148=CARTESIAN_POINT('Ctrl Pts',(-54.9426665516143,-2.95192631073098,
176.218540695264));
#13149=CARTESIAN_POINT('Ctrl Pts',(-54.9070365263685,-2.90171640292054,
176.413787336324));
#13150=CARTESIAN_POINT('Ctrl Pts',(-54.8013987998623,-2.81782847468563,
176.681821034794));
#13151=CARTESIAN_POINT('Ctrl Pts',(-54.7570848510793,-2.78787367953458,
176.767627228561));
#13152=CARTESIAN_POINT('Ctrl Pts',(-54.6793253219128,-2.74078668455889,
176.887592985838));
#13153=CARTESIAN_POINT('Ctrl Pts',(-54.651529701944,-2.72473899696222,176.926133356148));
#13154=CARTESIAN_POINT('Ctrl Pts',(-54.5925997439423,-2.69209575899625,
176.999824075839));
#13155=CARTESIAN_POINT('Ctrl Pts',(-54.5641015373143,-2.67654794454284,
177.031971691023));
#13156=CARTESIAN_POINT('Ctrl Pts',(-54.5288628436534,-2.65870383148503,
177.068203177065));
#13157=CARTESIAN_POINT('Ctrl Pts',(-49.7605161567837,-28.8447111186158,
177.498294784826));
#13158=CARTESIAN_POINT('Ctrl Pts',(-49.703499066658,-28.8235655424673,177.540214005203));
#13159=CARTESIAN_POINT('Ctrl Pts',(-49.6410455761305,-28.7951782353542,
177.600452889938));
#13160=CARTESIAN_POINT('Ctrl Pts',(-49.5125749804916,-28.7439261033728,
177.690427833332));
#13161=CARTESIAN_POINT('Ctrl Pts',(-49.4455382815264,-28.7177519743038,
177.731297783696));
#13162=CARTESIAN_POINT('Ctrl Pts',(-49.2376911387288,-28.6378112833129,
177.840935439774));
#13163=CARTESIAN_POINT('Ctrl Pts',(-49.0899159828253,-28.5824382846613,
177.897035937477));
#13164=CARTESIAN_POINT('Ctrl Pts',(-48.6337896696199,-28.4146446752159,
178.002589339604));
#13165=CARTESIAN_POINT('Ctrl Pts',(-48.3132270959126,-28.2997217083806,
177.992428880102));
#13166=CARTESIAN_POINT('Ctrl Pts',(-47.4162097247782,-27.9673749676665,
177.725331904959));
#13167=CARTESIAN_POINT('Ctrl Pts',(-46.9189492851719,-27.7652251395226,
177.218083285283));
#13168=CARTESIAN_POINT('Ctrl Pts',(-46.5632291525645,-27.4820421855238,
175.966063107167));
#13169=CARTESIAN_POINT('Ctrl Pts',(-46.7140098167225,-27.4055520605101,
175.249184591433));
#13170=CARTESIAN_POINT('Ctrl Pts',(-47.566085933826,-27.3558389712614,174.223160308952));
#13171=CARTESIAN_POINT('Ctrl Pts',(-48.2470586621674,-27.3810915115113,
173.939995635501));
#13172=CARTESIAN_POINT('Ctrl Pts',(-49.5700361455588,-27.4220834505067,
174.062399212278));
#13173=CARTESIAN_POINT('Ctrl Pts',(-50.1884067287968,-27.434811958294,174.470377906696));
#13174=CARTESIAN_POINT('Ctrl Pts',(-50.8303308863031,-27.3468909642006,
175.620618298056));
#13175=CARTESIAN_POINT('Ctrl Pts',(-50.8493116919004,-27.2434061722865,
176.356125167609));
#13176=CARTESIAN_POINT('Ctrl Pts',(-50.2816569479994,-26.9206929510016,
177.507808537998));
#13177=CARTESIAN_POINT('Ctrl Pts',(-49.6987348616025,-26.7015350212598,
177.912925525668));
#13178=CARTESIAN_POINT('Ctrl Pts',(-48.454710251186,-26.2485207329848,178.028292067179));
#13179=CARTESIAN_POINT('Ctrl Pts',(-47.8121824616331,-26.017945810327,177.739239128205));
#13180=CARTESIAN_POINT('Ctrl Pts',(-47.0491566977328,-25.6568136786021,
176.713556301102));
#13181=CARTESIAN_POINT('Ctrl Pts',(-46.9415518318806,-25.5298970910749,
175.993584668982));
#13182=CARTESIAN_POINT('Ctrl Pts',(-47.3778834474909,-25.4016448622981,
174.749674324357));
#13183=CARTESIAN_POINT('Ctrl Pts',(-47.9149438708112,-25.3989201973124,
174.243242130538));
#13184=CARTESIAN_POINT('Ctrl Pts',(-49.195098595239,-25.4317364372956,173.888113334518));
#13185=CARTESIAN_POINT('Ctrl Pts',(-49.918185567551,-25.4646653275392,174.050133776974));
#13186=CARTESIAN_POINT('Ctrl Pts',(-50.9295131393841,-25.4466210128473,
174.911633886668));
#13187=CARTESIAN_POINT('Ctrl Pts',(-51.2044913533823,-25.3930064438348,
175.597822621196));
#13188=CARTESIAN_POINT('Ctrl Pts',(-51.0754639563939,-25.1539869007477,
176.899089439364));
#13189=CARTESIAN_POINT('Ctrl Pts',(-50.6742118208058,-24.9705041413757,
177.491449801663));
#13190=CARTESIAN_POINT('Ctrl Pts',(-49.5587075034334,-24.5430242840169,
178.062955652865));
#13191=CARTESIAN_POINT('Ctrl Pts',(-48.8611723259578,-24.3021716495128,
178.034645386427));
#13192=CARTESIAN_POINT('Ctrl Pts',(-47.7896195282427,-23.8814983836082,
177.370866230542));
#13193=CARTESIAN_POINT('Ctrl Pts',(-47.4363508410467,-23.7069028048269,
176.742728542957));
#13194=CARTESIAN_POINT('Ctrl Pts',(-47.4114253180649,-23.4889969329168,
175.432113003805));
#13195=CARTESIAN_POINT('Ctrl Pts',(-47.740070725129,-23.4456714422117,174.768834597493));
#13196=CARTESIAN_POINT('Ctrl Pts',(-48.8702204177861,-23.4389819923271,
173.952056567371));
#13197=CARTESIAN_POINT('Ctrl Pts',(-49.6947930376395,-23.4814638927378,
173.877925688461));
#13198=CARTESIAN_POINT('Ctrl Pts',(-51.0112605873021,-23.5013279450334,
174.502758507842));
#13199=CARTESIAN_POINT('Ctrl Pts',(-51.4766740890821,-23.4736078700863,
175.190881305064));
#13200=CARTESIAN_POINT('Ctrl Pts',(-51.5715098854918,-23.2578265151817,
176.631332013987));
#13201=CARTESIAN_POINT('Ctrl Pts',(-51.2026984232359,-23.0689810535093,
177.353708555585));
#13202=CARTESIAN_POINT('Ctrl Pts',(-50.0169981786826,-22.6055963153184,
178.072791197941));
#13203=CARTESIAN_POINT('Ctrl Pts',(-49.2289032454779,-22.3364394885883,
178.054791801573));
#13204=CARTESIAN_POINT('Ctrl Pts',(-48.0752306219957,-21.8785657833076,
177.283552800795));
#13205=CARTESIAN_POINT('Ctrl Pts',(-47.7373875210752,-21.6968802590999,
176.548566639058));
#13206=CARTESIAN_POINT('Ctrl Pts',(-47.8901343487967,-21.492320838371,175.113663385513));
#13207=CARTESIAN_POINT('Ctrl Pts',(-48.3804128007365,-21.4693940830233,
174.442825661914));
#13208=CARTESIAN_POINT('Ctrl Pts',(-49.7230759786915,-21.4942443138953,
173.870938911605));
#13209=CARTESIAN_POINT('Ctrl Pts',(-50.5477501626655,-21.53554466513,173.979304242753));
#13210=CARTESIAN_POINT('Ctrl Pts',(-51.6956775721548,-21.5221965965903,
174.884495307656));
#13211=CARTESIAN_POINT('Ctrl Pts',(-51.995185395164,-21.4627711751308,175.65946330393));
#13212=CARTESIAN_POINT('Ctrl Pts',(-51.7684808698132,-21.1836626405178,
177.075777271268));
#13213=CARTESIAN_POINT('Ctrl Pts',(-51.248410167092,-20.9668436684778,177.683928269078));
#13214=CARTESIAN_POINT('Ctrl Pts',(-49.9393032270381,-20.4803392816045,
178.101596183419));
#13215=CARTESIAN_POINT('Ctrl Pts',(-49.1773119956809,-20.2159303489599,
177.900701030808));
#13216=CARTESIAN_POINT('Ctrl Pts',(-48.2258296454727,-19.7984008812386,
176.875814996871));
#13217=CARTESIAN_POINT('Ctrl Pts',(-48.0552229745052,-19.6477554978605,
176.074637438704));
#13218=CARTESIAN_POINT('Ctrl Pts',(-48.5258258225559,-19.5038059294262,
174.698094313544));
#13219=CARTESIAN_POINT('Ctrl Pts',(-49.1555523948045,-19.5080820109078,
174.15313676254));
#13220=CARTESIAN_POINT('Ctrl Pts',(-50.5933891726929,-19.5499376382275,
173.895161972129));
#13221=CARTESIAN_POINT('Ctrl Pts',(-51.368058411907,-19.5828296420673,174.188177381599));
#13222=CARTESIAN_POINT('Ctrl Pts',(-52.285250485287,-19.5255903568737,175.320127767442));
#13223=CARTESIAN_POINT('Ctrl Pts',(-52.4079017329002,-19.4317611692977,
176.136959370172));
#13224=CARTESIAN_POINT('Ctrl Pts',(-51.8753008807154,-19.0950488584311,
177.453114298066));
#13225=CARTESIAN_POINT('Ctrl Pts',(-51.2342686483785,-18.8536936439763,
177.926872571079));
#13226=CARTESIAN_POINT('Ctrl Pts',(-49.8632157867063,-18.3545541183897,
178.021760725256));
#13227=CARTESIAN_POINT('Ctrl Pts',(-49.1660096364335,-18.1030331017558,
177.643137201611));
#13228=CARTESIAN_POINT('Ctrl Pts',(-48.4670297183309,-17.7327410070788,
176.413682699456));
#13229=CARTESIAN_POINT('Ctrl Pts',(-48.483334940274,-17.6194284897493,175.592916154309));
#13230=CARTESIAN_POINT('Ctrl Pts',(-49.2450668681383,-17.5322013902257,
174.352697167155));
#13231=CARTESIAN_POINT('Ctrl Pts',(-49.9777722871607,-17.5559821453049,
173.960304681794));
#13232=CARTESIAN_POINT('Ctrl Pts',(-51.4344516507071,-17.6029063882428,
174.028937019837));
#13233=CARTESIAN_POINT('Ctrl Pts',(-52.1305828574604,-17.6193975644539,
174.485906049309));
#13234=CARTESIAN_POINT('Ctrl Pts',(-52.774838706301,-17.5089074046146,175.793694056009));
#13235=CARTESIAN_POINT('Ctrl Pts',(-52.7115258732458,-17.3796686755426,
176.613178448276));
#13236=CARTESIAN_POINT('Ctrl Pts',(-51.9002446822929,-16.9876585431162,
177.764926590858));
#13237=CARTESIAN_POINT('Ctrl Pts',(-51.1728057089079,-16.7309097600974,
178.068009087089));
#13238=CARTESIAN_POINT('Ctrl Pts',(-49.8211348979667,-16.2361848829689,
177.837068581403));
#13239=CARTESIAN_POINT('Ctrl Pts',(-49.2256314668982,-16.0038069200319,
177.305047152795));
#13240=CARTESIAN_POINT('Ctrl Pts',(-48.8186328386387,-15.691330495564,175.939125806104));
#13241=CARTESIAN_POINT('Ctrl Pts',(-49.013546517339,-15.6112127223192,175.133605172695));
#13242=CARTESIAN_POINT('Ctrl Pts',(-50.0357499087345,-15.5735396207079,
174.088389632472));
#13243=CARTESIAN_POINT('Ctrl Pts',(-50.8379174497137,-15.6112366284576,
173.871670522767));
#13244=CARTESIAN_POINT('Ctrl Pts',(-52.2457834487726,-15.6472027358935,
174.26447248136));
#13245=CARTESIAN_POINT('Ctrl Pts',(-52.8170337247495,-15.6408479370702,
174.8653310014));
#13246=CARTESIAN_POINT('Ctrl Pts',(-53.1560440051794,-15.4721566908598,
176.273031298879));
#13247=CARTESIAN_POINT('Ctrl Pts',(-52.9154253174859,-15.3082073561117,
177.052126824288));
#13248=CARTESIAN_POINT('Ctrl Pts',(-51.8728096300678,-14.8731360568539,
177.975770830197));
#13249=CARTESIAN_POINT('Ctrl Pts',(-51.0951645133176,-14.6055143185424,
178.104087436367));
#13250=CARTESIAN_POINT('Ctrl Pts',(-49.8271933090145,-14.1262171391814,
177.555333624295));
#13251=CARTESIAN_POINT('Ctrl Pts',(-49.3671436709228,-13.9204374671742,
176.893150416479));
#13252=CARTESIAN_POINT('Ctrl Pts',(-49.274728926638,-13.6672296225191,175.457007277905));
#13253=CARTESIAN_POINT('Ctrl Pts',(-49.6465886024413,-13.6223148063404,
174.716642572685));
#13254=CARTESIAN_POINT('Ctrl Pts',(-50.8704338551746,-13.6242867085274,
173.925061362222));
#13255=CARTESIAN_POINT('Ctrl Pts',(-51.7000786840932,-13.666773744136,173.890948850678));
#13256=CARTESIAN_POINT('Ctrl Pts',(-52.983493848767,-13.6801901085456,174.58610021153));
#13257=CARTESIAN_POINT('Ctrl Pts',(-53.4130967944053,-13.6453172862449,
175.298527478907));
#13258=CARTESIAN_POINT('Ctrl Pts',(-53.4312271360186,-13.4141834163833,
176.741466379681));
#13259=CARTESIAN_POINT('Ctrl Pts',(-53.0223631213944,-13.2182197961852,
177.439586265974));
#13260=CARTESIAN_POINT('Ctrl Pts',(-51.8015717929752,-12.7473718779738,
178.090703687822));
#13261=CARTESIAN_POINT('Ctrl Pts',(-51.0193050555008,-12.4800112867217,
178.027617006182));
#13262=CARTESIAN_POINT('Ctrl Pts',(-49.9091230827754,-12.0317475039094,
177.194798446979));
#13263=CARTESIAN_POINT('Ctrl Pts',(-49.6065982226317,-11.8558917537395,
176.440442987632));
#13264=CARTESIAN_POINT('Ctrl Pts',(-49.8356019855053,-11.6660764580159,
175.012059004046));
#13265=CARTESIAN_POINT('Ctrl Pts',(-50.3610430198266,-11.6496605652263,
174.366149315963));
#13266=CARTESIAN_POINT('Ctrl Pts',(-51.7343806490719,-11.6797988495863,
173.866104995302));
#13267=CARTESIAN_POINT('Ctrl Pts',(-52.550540790582,-11.7201981252995,174.02088411371));
#13268=CARTESIAN_POINT('Ctrl Pts',(-53.6500640270725,-11.6966559909963,
174.984749041133));
#13269=CARTESIAN_POINT('Ctrl Pts',(-53.9056865612328,-11.6294298688172,
175.770695352483));
#13270=CARTESIAN_POINT('Ctrl Pts',(-53.6065172861421,-11.3376692947806,
177.167270913611));
#13271=CARTESIAN_POINT('Ctrl Pts',(-53.0559160748103,-11.1139055956972,
177.749439639131));
#13272=CARTESIAN_POINT('Ctrl Pts',(-51.7252371686403,-10.6233177496803,
178.092170345976));
#13273=CARTESIAN_POINT('Ctrl Pts',(-50.9736524019596,-10.3607126008384,
177.849203208466));
#13274=CARTESIAN_POINT('Ctrl Pts',(-50.0765013772471,-9.95292884744916,
176.76875224789));
#13275=CARTESIAN_POINT('Ctrl Pts',(-49.9516819265813,-9.81183425780667,
175.958513771998));
#13276=CARTESIAN_POINT('Ctrl Pts',(-50.4932223958658,-9.68088414604229,
174.607725553029));
#13277=CARTESIAN_POINT('Ctrl Pts',(-51.1493491071183,-9.69075789692425,
174.099564788001));
#13278=CARTESIAN_POINT('Ctrl Pts',(-52.5949212007306,-9.73546275490891,
173.917493057606));
#13279=CARTESIAN_POINT('Ctrl Pts',(-53.3569613223681,-9.76490646019358,
174.248860303054));
#13280=CARTESIAN_POINT('Ctrl Pts',(-54.2135986647274,-9.69602761498083,
175.428657754819));
#13281=CARTESIAN_POINT('Ctrl Pts',(-54.293848370144,-9.59379233086061,176.251060243097));
#13282=CARTESIAN_POINT('Ctrl Pts',(-53.6913007216372,-9.24298063305673,
177.535379997424));
#13283=CARTESIAN_POINT('Ctrl Pts',(-53.0251793740895,-8.99747173235245,
177.96924977839));
#13284=CARTESIAN_POINT('Ctrl Pts',(-51.651725273033,-8.49712492600163,177.987723094373));
#13285=CARTESIAN_POINT('Ctrl Pts',(-50.9786512815054,-8.25081939601668,
177.570771429869));
#13286=CARTESIAN_POINT('Ctrl Pts',(-50.3458167934762,-7.89459730610716,
176.305935969218));
#13287=CARTESIAN_POINT('Ctrl Pts',(-50.4021522245058,-7.78795543802409,
175.483191418641));
#13288=CARTESIAN_POINT('Ctrl Pts',(-51.2295886328818,-7.71347110197539,
174.283262770515));
#13289=CARTESIAN_POINT('Ctrl Pts',(-51.9823539758956,-7.74096536711586,
173.929068927273));
#13290=CARTESIAN_POINT('Ctrl Pts',(-53.4363603166253,-7.78662015021704,
174.075813689628));
#13291=CARTESIAN_POINT('Ctrl Pts',(-54.1043459363082,-7.79847651244032,
174.570723179108));
#13292=CARTESIAN_POINT('Ctrl Pts',(-54.6799658608561,-7.67397811007903,
175.90877571489));
#13293=CARTESIAN_POINT('Ctrl Pts',(-54.5722464428634,-7.53659878310187,
176.719948913595));
#13294=CARTESIAN_POINT('Ctrl Pts',(-53.7048106882453,-7.13527023180301,
177.820508243663));
#13295=CARTESIAN_POINT('Ctrl Pts',(-52.9613211614002,-6.87434685741961,
178.086941994317));
#13296=CARTESIAN_POINT('Ctrl Pts',(-51.6221407922901,-6.38201846097514,
177.778890662373));
#13297=CARTESIAN_POINT('Ctrl Pts',(-51.0546870579556,-6.15491662175662,
177.213869145202));
#13298=CARTESIAN_POINT('Ctrl Pts',(-50.7203127232504,-5.85585141799114,
175.823263107997));
#13299=CARTESIAN_POINT('Ctrl Pts',(-50.9602054908589,-5.78500310757108,
175.029480964866));
#13300=CARTESIAN_POINT('Ctrl Pts',(-52.0343424634976,-5.75674450428783,
174.039165918607));
#13301=CARTESIAN_POINT('Ctrl Pts',(-52.8447329543179,-5.79646505952858,
173.866867743832));
#13302=CARTESIAN_POINT('Ctrl Pts',(-54.227093102642,-5.82880399980787,174.331684606762));
#13303=CARTESIAN_POINT('Ctrl Pts',(-54.7703330160768,-5.81603743040407,
174.961265757845));
#13304=CARTESIAN_POINT('Ctrl Pts',(-55.0342584322448,-5.63295034503888,
176.384531023624));
#13305=CARTESIAN_POINT('Ctrl Pts',(-54.7535167216846,-5.46110103683509,
177.149304158576));
#13306=CARTESIAN_POINT('Ctrl Pts',(-53.6617191466184,-5.01587299208642,
178.013397713687));
#13307=CARTESIAN_POINT('Ctrl Pts',(-52.8789563910228,-4.7479816344422,178.094733745787));
#13308=CARTESIAN_POINT('Ctrl Pts',(-51.6416463903481,-4.27383996939189,
177.476508505419));
#13309=CARTESIAN_POINT('Ctrl Pts',(-51.2194660036301,-4.07584859930261,
176.790317421121));
#13310=CARTESIAN_POINT('Ctrl Pts',(-51.2019938075703,-3.83837584139065,
175.351935740118));
#13311=CARTESIAN_POINT('Ctrl Pts',(-51.610208243602,-3.79954787084599,174.628251672824));
#13312=CARTESIAN_POINT('Ctrl Pts',(-52.8762543405249,-3.80961476365013,
173.901884637809));
#13313=CARTESIAN_POINT('Ctrl Pts',(-53.7073988028502,-3.85223555101975,
173.911595161346));
#13314=CARTESIAN_POINT('Ctrl Pts',(-54.9534921954892,-3.85792953287916,
174.67446559102));
#13315=CARTESIAN_POINT('Ctrl Pts',(-55.3426629917145,-3.81570008082077,
175.409213860003));
#13316=CARTESIAN_POINT('Ctrl Pts',(-55.3039033258818,-3.64772468214507,
176.391662012851));
#13317=CARTESIAN_POINT('Ctrl Pts',(-55.240555748585,-3.59330136077634,176.648581151648));
#13318=CARTESIAN_POINT('Ctrl Pts',(-55.0788320999402,-3.49759375703432,
177.001372563377));
#13319=CARTESIAN_POINT('Ctrl Pts',(-55.0131335998823,-3.46357400887706,
177.112553347482));
#13320=CARTESIAN_POINT('Ctrl Pts',(-54.8999581434668,-3.40984365170443,
177.267014142137));
#13321=CARTESIAN_POINT('Ctrl Pts',(-54.8598034384417,-3.39148030846876,
177.316464483235));
#13322=CARTESIAN_POINT('Ctrl Pts',(-54.7750771562006,-3.35389509449369,
177.410924972696));
#13323=CARTESIAN_POINT('Ctrl Pts',(-54.7397209311609,-3.33918794957438,
177.445275075635));
#13324=CARTESIAN_POINT('Ctrl Pts',(-54.6838989306507,-3.31503673670408,
177.498541333932));
#13325=CARTESIAN_POINT('Ctrl Pts',(-50.3479071748434,-28.4569951884828,
177.87862115707));
#13326=CARTESIAN_POINT('Ctrl Pts',(-50.2728575672733,-28.4359962578257,
177.948540001849));
#13327=CARTESIAN_POINT('Ctrl Pts',(-50.1962258409275,-28.4010191615162,
178.021251708215));
#13328=CARTESIAN_POINT('Ctrl Pts',(-50.0327133344336,-28.3431284715803,
178.148112768101));
#13329=CARTESIAN_POINT('Ctrl Pts',(-49.9471957757512,-28.3135226108735,
178.206264690109));
#13330=CARTESIAN_POINT('Ctrl Pts',(-49.6807194301921,-28.2224721023673,
178.364232700982));
#13331=CARTESIAN_POINT('Ctrl Pts',(-49.4886308694229,-28.1579103591893,
178.447943211646));
#13332=CARTESIAN_POINT('Ctrl Pts',(-48.8935956196606,-27.9633647516093,
178.618732735728));
#13333=CARTESIAN_POINT('Ctrl Pts',(-48.4698811368596,-27.8285932845993,
178.628088311833));
#13334=CARTESIAN_POINT('Ctrl Pts',(-47.2704244122812,-27.4388125604887,
178.343093993075));
#13335=CARTESIAN_POINT('Ctrl Pts',(-46.5780488855805,-27.1997688494767,
177.716319207522));
#13336=CARTESIAN_POINT('Ctrl Pts',(-46.0180477417519,-26.8743979377982,
176.099249510754));
#13337=CARTESIAN_POINT('Ctrl Pts',(-46.162624656611,-26.7973830650002,175.153557109113));
#13338=CARTESIAN_POINT('Ctrl Pts',(-47.1953010051746,-26.7839304768722,
173.755742992678));
#13339=CARTESIAN_POINT('Ctrl Pts',(-48.0607153645256,-26.8454387863112,
173.337748493251));
#13340=CARTESIAN_POINT('Ctrl Pts',(-49.7936242958811,-26.9626978867657,
173.412243144396));
#13341=CARTESIAN_POINT('Ctrl Pts',(-50.6218862360795,-27.016572452629,173.905326198308));
#13342=CARTESIAN_POINT('Ctrl Pts',(-51.5258205855669,-26.9805930176338,
175.367177784907));
#13343=CARTESIAN_POINT('Ctrl Pts',(-51.5951438365624,-26.8874613833773,
176.329869003407));
#13344=CARTESIAN_POINT('Ctrl Pts',(-50.9127162462792,-26.5399486517808,
177.882574589842));
#13345=CARTESIAN_POINT('Ctrl Pts',(-50.1707795944383,-26.2907274748939,
178.452449051012));
#13346=CARTESIAN_POINT('Ctrl Pts',(-48.5397246316051,-25.7645038790956,
178.692502082553));
#13347=CARTESIAN_POINT('Ctrl Pts',(-47.67260524551,-25.4913101058597,178.361691922331));
#13348=CARTESIAN_POINT('Ctrl Pts',(-46.5924693917267,-25.0662449204663,
177.069022085109));
#13349=CARTESIAN_POINT('Ctrl Pts',(-46.3991806471167,-24.9234731673228,
176.136653590829));
#13350=CARTESIAN_POINT('Ctrl Pts',(-46.8738389297659,-24.8040321200569,
174.482872284355));
#13351=CARTESIAN_POINT('Ctrl Pts',(-47.5355683392896,-24.8259889159373,
173.783025779917));
#13352=CARTESIAN_POINT('Ctrl Pts',(-49.181078144729,-24.926602323961,173.233424036193));
#13353=CARTESIAN_POINT('Ctrl Pts',(-50.130455303743,-25.0037631556439,173.398086820976));
#13354=CARTESIAN_POINT('Ctrl Pts',(-51.4978889309697,-25.0558147041254,
174.456799989093));
#13355=CARTESIAN_POINT('Ctrl Pts',(-51.8989353348306,-25.0272033256972,
175.336539369917));
#13356=CARTESIAN_POINT('Ctrl Pts',(-51.8018863283238,-24.7915666340119,
177.05629857501));
#13357=CARTESIAN_POINT('Ctrl Pts',(-51.3095767986978,-24.5911935663349,
177.858613821852));
#13358=CARTESIAN_POINT('Ctrl Pts',(-49.8771546536489,-24.10401978861,178.68604557473));
#13359=CARTESIAN_POINT('Ctrl Pts',(-48.9560458718938,-23.8206956072764,
178.700341600297));
#13360=CARTESIAN_POINT('Ctrl Pts',(-47.4944002604164,-23.3221357921539,
177.903717692127));
#13361=CARTESIAN_POINT('Ctrl Pts',(-46.9859140286074,-23.1182050059858,
177.107706307993));
#13362=CARTESIAN_POINT('Ctrl Pts',(-46.8530474021693,-22.8809089149922,
175.398792520737));
#13363=CARTESIAN_POINT('Ctrl Pts',(-47.231059536602,-22.8477944049951,174.508609012772));
#13364=CARTESIAN_POINT('Ctrl Pts',(-48.6493873331158,-22.8937567040743,
173.363150661036));
#13365=CARTESIAN_POINT('Ctrl Pts',(-49.7143921444323,-22.9840542321675,
173.211662996139));
#13366=CARTESIAN_POINT('Ctrl Pts',(-51.4652368913311,-23.0881428692961,
173.941607840096));
#13367=CARTESIAN_POINT('Ctrl Pts',(-52.1136094605607,-23.094525291844,174.813935779811));
#13368=CARTESIAN_POINT('Ctrl Pts',(-52.3204663109761,-22.9019098705719,
176.69350767169));
#13369=CARTESIAN_POINT('Ctrl Pts',(-51.877821743202,-22.6977464609932,177.66752824204));
#13370=CARTESIAN_POINT('Ctrl Pts',(-50.3601753662095,-22.1706433373772,
178.693383453661));
#13371=CARTESIAN_POINT('Ctrl Pts',(-49.3218325614145,-21.8547798388568,
178.72781114664));
#13372=CARTESIAN_POINT('Ctrl Pts',(-47.7441093775104,-21.3120724766084,
177.795709587611));
#13373=CARTESIAN_POINT('Ctrl Pts',(-47.2477760409393,-21.1012761066736,
176.860414332907));
#13374=CARTESIAN_POINT('Ctrl Pts',(-47.3387825873497,-20.8852685243919,
174.97505816188));
#13375=CARTESIAN_POINT('Ctrl Pts',(-47.9314309575524,-20.8809046965219,
174.063915635121));
#13376=CARTESIAN_POINT('Ctrl Pts',(-49.6347357453554,-20.9768646680186,
173.225964829082));
#13377=CARTESIAN_POINT('Ctrl Pts',(-50.7167240875825,-21.0667038014875,
173.313184970442));
#13378=CARTESIAN_POINT('Ctrl Pts',(-52.2657610285106,-21.1310010461024,
174.421840220958));
#13379=CARTESIAN_POINT('Ctrl Pts',(-52.7037384700293,-21.0998274566763,
175.41493210957));
#13380=CARTESIAN_POINT('Ctrl Pts',(-52.4847175837037,-20.8191405044519,
177.292562937125));
#13381=CARTESIAN_POINT('Ctrl Pts',(-51.8386241308113,-20.5794725658491,
178.12361350116));
#13382=CARTESIAN_POINT('Ctrl Pts',(-50.1396663396365,-20.018246073474,178.763454537015));
#13383=CARTESIAN_POINT('Ctrl Pts',(-49.1209540205185,-19.7031542981699,
178.552891694314));
#13384=CARTESIAN_POINT('Ctrl Pts',(-47.794702927651,-19.2149188701855,177.282197399313));
#13385=CARTESIAN_POINT('Ctrl Pts',(-47.5115450575125,-19.0414866308731,
176.244710688925));
#13386=CARTESIAN_POINT('Ctrl Pts',(-48.0225076992042,-18.9056180257745,
174.413639337664));
#13387=CARTESIAN_POINT('Ctrl Pts',(-48.8010517900779,-18.9401402740231,
173.657816206187));
#13388=CARTESIAN_POINT('Ctrl Pts',(-50.6589325202962,-19.0599362479824,
173.225466551806));
#13389=CARTESIAN_POINT('Ctrl Pts',(-51.6828783925415,-19.1423524153639,
173.556811131415));
#13390=CARTESIAN_POINT('Ctrl Pts',(-52.94490571859,-19.1520660317591,174.977944054317));
#13391=CARTESIAN_POINT('Ctrl Pts',(-53.1522316495948,-19.0733891332466,
176.042129261136));
#13392=CARTESIAN_POINT('Ctrl Pts',(-52.5304975170958,-18.7210523123868,
177.802820234119));
#13393=CARTESIAN_POINT('Ctrl Pts',(-51.7144732100097,-18.4448678812944,
178.469420248747));
#13394=CARTESIAN_POINT('Ctrl Pts',(-49.9127782169188,-17.8629843097264,
178.691085462265));
#13395=CARTESIAN_POINT('Ctrl Pts',(-48.9683571282271,-17.5653381811437,
178.247635108413));
#13396=CARTESIAN_POINT('Ctrl Pts',(-47.9579076603942,-17.1319211116872,
176.683402031933));
#13397=CARTESIAN_POINT('Ctrl Pts',(-47.9184077060768,-17.009302655329,175.611974434002));
#13398=CARTESIAN_POINT('Ctrl Pts',(-48.8193204272181,-16.9493687678545,
173.939410793842));
#13399=CARTESIAN_POINT('Ctrl Pts',(-49.7479148095836,-17.0097492793151,
173.377008912436));
#13400=CARTESIAN_POINT('Ctrl Pts',(-51.643208967551,-17.1428193004232,173.368498519432));
#13401=CARTESIAN_POINT('Ctrl Pts',(-52.5796094505093,-17.2045582837911,
173.921665784702));
#13402=CARTESIAN_POINT('Ctrl Pts',(-53.4961681928706,-17.1468816411331,
175.591939966795));
#13403=CARTESIAN_POINT('Ctrl Pts',(-53.4629851797616,-17.024999612415,176.669185388437));
#13404=CARTESIAN_POINT('Ctrl Pts',(-52.4593346223015,-16.5928308404044,
178.238747171052));
#13405=CARTESIAN_POINT('Ctrl Pts',(-51.5224253668316,-16.2971453030902,
178.685547111838));
#13406=CARTESIAN_POINT('Ctrl Pts',(-49.7246467734476,-15.7168449309467,
178.479497386489));
#13407=CARTESIAN_POINT('Ctrl Pts',(-48.9027009029283,-15.4396261238498,
177.823563805929));
#13408=CARTESIAN_POINT('Ctrl Pts',(-48.2654141259822,-15.0843052308904,
176.069175886686));
#13409=CARTESIAN_POINT('Ctrl Pts',(-48.4613159716259,-15.0032908855178,
175.000998038449));
#13410=CARTESIAN_POINT('Ctrl Pts',(-49.7162174501553,-15.01079667333,173.565578406105));
#13411=CARTESIAN_POINT('Ctrl Pts',(-50.7428205977302,-15.0933182852754,
173.226451476554));
#13412=CARTESIAN_POINT('Ctrl Pts',(-52.6035006910652,-15.2135426682566,
173.650512878487));
#13413=CARTESIAN_POINT('Ctrl Pts',(-53.382025542189,-15.2486168447941,174.397702687793));
#13414=CARTESIAN_POINT('Ctrl Pts',(-53.905727267535,-15.1159903036539,176.219573585739));
#13415=CARTESIAN_POINT('Ctrl Pts',(-53.6343010604909,-14.9449274325696,
177.258764585683));
#13416=CARTESIAN_POINT('Ctrl Pts',(-52.3195045847479,-14.4589334435455,
178.541768722646));
#13417=CARTESIAN_POINT('Ctrl Pts',(-51.3015568868895,-14.1438839803641,
178.764698457169));
#13418=CARTESIAN_POINT('Ctrl Pts',(-49.5920248617255,-13.5797433288121,
178.136857041975));
#13419=CARTESIAN_POINT('Ctrl Pts',(-48.9380275082558,-13.3381062047143,
177.30578604004));
#13420=CARTESIAN_POINT('Ctrl Pts',(-48.7105476579708,-13.0557925005452,
175.429441731563));
#13421=CARTESIAN_POINT('Ctrl Pts',(-49.1406103931943,-13.0235604552581,
174.438788862592));
#13422=CARTESIAN_POINT('Ctrl Pts',(-50.6761207099769,-13.0860799668151,
173.321489243126));
#13423=CARTESIAN_POINT('Ctrl Pts',(-51.7550963134731,-13.1754760058423,
173.222308149713));
#13424=CARTESIAN_POINT('Ctrl Pts',(-53.4658619993328,-13.2728668841322,
174.044907498799));
#13425=CARTESIAN_POINT('Ctrl Pts',(-54.0695830139971,-13.2704822339251,
174.951304580462));
#13426=CARTESIAN_POINT('Ctrl Pts',(-54.1756431350045,-13.0566118191168,
176.841599266944));
#13427=CARTESIAN_POINT('Ctrl Pts',(-53.682402379201,-12.8459201272062,177.784941606983));
#13428=CARTESIAN_POINT('Ctrl Pts',(-52.1086906323698,-12.3039548020853,
178.724742549594));
#13429=CARTESIAN_POINT('Ctrl Pts',(-51.0761365726385,-11.9897880340734,
178.697123202695));
#13430=CARTESIAN_POINT('Ctrl Pts',(-49.5543778605173,-11.4626036611189,
177.68675201361));
#13431=CARTESIAN_POINT('Ctrl Pts',(-49.102117382649,-11.2567014833508,176.719561205716));
#13432=CARTESIAN_POINT('Ctrl Pts',(-49.292107286816,-11.0609269687249,174.839303437302));
#13433=CARTESIAN_POINT('Ctrl Pts',(-49.9319808722111,-11.065488255827,173.957841233623));
#13434=CARTESIAN_POINT('Ctrl Pts',(-51.6826661337304,-11.1687038756892,
173.21175444078));
#13435=CARTESIAN_POINT('Ctrl Pts',(-52.7531972098707,-11.2596980870477,
173.357216390535));
#13436=CARTESIAN_POINT('Ctrl Pts',(-54.2460458385202,-11.3089418781751,
174.551734842451));
#13437=CARTESIAN_POINT('Ctrl Pts',(-54.6245671161656,-11.2668768405657,
175.56211463078));
#13438=CARTESIAN_POINT('Ctrl Pts',(-54.3123472668563,-10.9730441873765,
177.413426209709));
#13439=CARTESIAN_POINT('Ctrl Pts',(-53.6216949876352,-10.7211032153202,
178.215314744748));
#13440=CARTESIAN_POINT('Ctrl Pts',(-51.8913746121094,-10.1550133368813,
178.758899998487));
#13441=CARTESIAN_POINT('Ctrl Pts',(-50.8831280746124,-9.84182247697009,
178.493145848044));
#13442=CARTESIAN_POINT('Ctrl Pts',(-49.6236112332636,-9.36447275925141,
177.143870489208));
#13443=CARTESIAN_POINT('Ctrl Pts',(-49.3975849797945,-9.20540142615231,
176.095279478262));
#13444=CARTESIAN_POINT('Ctrl Pts',(-50.0079456983536,-9.08466255147406,
174.288405253537));
#13445=CARTESIAN_POINT('Ctrl Pts',(-50.8244602905949,-9.12692713822202,
173.581609594638));
#13446=CARTESIAN_POINT('Ctrl Pts',(-52.6906598209441,-9.25318698046637,
173.246687842459));
#13447=CARTESIAN_POINT('Ctrl Pts',(-53.7047460872083,-9.33006604421617,
173.631253257821));
#13448=CARTESIAN_POINT('Ctrl Pts',(-54.8900559939021,-9.32613298909108,
175.117109460381));
#13449=CARTESIAN_POINT('Ctrl Pts',(-55.0428852800419,-9.23680213120813,
176.191613835385));
#13450=CARTESIAN_POINT('Ctrl Pts',(-54.3260630027991,-8.86426623816917,
177.917066297754));
#13451=CARTESIAN_POINT('Ctrl Pts',(-53.4783261791472,-8.5852751826903,178.533414961083));
#13452=CARTESIAN_POINT('Ctrl Pts',(-51.6632029807945,-7.99669600625119,
178.652882987613));
#13453=CARTESIAN_POINT('Ctrl Pts',(-50.7499980781025,-7.70554604519678,
178.155739114359));
#13454=CARTESIAN_POINT('Ctrl Pts',(-49.8242259537338,-7.29327695933862,
176.547077701437));
#13455=CARTESIAN_POINT('Ctrl Pts',(-49.838033268214,-7.17726487827271,175.466032067978));
#13456=CARTESIAN_POINT('Ctrl Pts',(-50.8256764893838,-7.13523953214819,
173.842841571287));
#13457=CARTESIAN_POINT('Ctrl Pts',(-51.7828991970818,-7.20106754009712,
173.328393136411));
#13458=CARTESIAN_POINT('Ctrl Pts',(-53.682121466631,-7.33289296119618,173.423267613666));
#13459=CARTESIAN_POINT('Ctrl Pts',(-54.5824458512144,-7.39109185214275,
174.023927494841));
#13460=CARTESIAN_POINT('Ctrl Pts',(-55.4117106483233,-7.31244449093335,
175.744908515432));
#13461=CARTESIAN_POINT('Ctrl Pts',(-55.3174225063257,-7.17911919393448,
176.81298142285));
#13462=CARTESIAN_POINT('Ctrl Pts',(-54.241836216539,-6.73809069114013,178.316074643566));
#13463=CARTESIAN_POINT('Ctrl Pts',(-53.2777666803375,-6.43346338348791,
178.716995563853));
#13464=CARTESIAN_POINT('Ctrl Pts',(-51.492709987459,-5.85671796076922,178.410389321177));
#13465=CARTESIAN_POINT('Ctrl Pts',(-50.7047045568934,-5.58599179870949,
177.709705935534));
#13466=CARTESIAN_POINT('Ctrl Pts',(-50.1611589540997,-5.24690475917716,
175.91572047402));
#13467=CARTESIAN_POINT('Ctrl Pts',(-50.412988668319,-5.17989675417243,174.862537959116));
#13468=CARTESIAN_POINT('Ctrl Pts',(-51.7459369624996,-5.19848686371817,
173.493142781303));
#13469=CARTESIAN_POINT('Ctrl Pts',(-52.7859565461007,-5.28395186106844,
173.214419006065));
#13470=CARTESIAN_POINT('Ctrl Pts',(-54.6124153348595,-5.40237052054082,
173.730440016312));
#13471=CARTESIAN_POINT('Ctrl Pts',(-55.3590089692939,-5.42765093815174,
174.520747942326));
#13472=CARTESIAN_POINT('Ctrl Pts',(-55.7857743262001,-5.27753030569205,
176.366096056906));
#13473=CARTESIAN_POINT('Ctrl Pts',(-55.461398252989,-5.09617167994865,177.38970404608));
#13474=CARTESIAN_POINT('Ctrl Pts',(-54.0763289367501,-4.5947076574371,178.59887213214));
#13475=CARTESIAN_POINT('Ctrl Pts',(-53.0518069694618,-4.2817330879142,178.762764238352));
#13476=CARTESIAN_POINT('Ctrl Pts',(-51.3741810061549,-3.71961935803744,
178.037173193724));
#13477=CARTESIAN_POINT('Ctrl Pts',(-50.7709128345885,-3.48817293681553,
177.171361011829));
#13478=CARTESIAN_POINT('Ctrl Pts',(-50.6389382081356,-3.22905679794207,
175.293151941354));
#13479=CARTESIAN_POINT('Ctrl Pts',(-51.12053621277,-3.20321300476925,174.318272388974));
#13480=CARTESIAN_POINT('Ctrl Pts',(-52.7133196362096,-3.27785561089881,
173.283689189228));
#13481=CARTESIAN_POINT('Ctrl Pts',(-53.7973395798457,-3.36818712000785,
173.24106430149));
#13482=CARTESIAN_POINT('Ctrl Pts',(-55.4653436163453,-3.45546685002776,
174.15674387015));
#13483=CARTESIAN_POINT('Ctrl Pts',(-56.0173052873986,-3.44570666511222,
175.091057375796));
#13484=CARTESIAN_POINT('Ctrl Pts',(-56.0215539606611,-3.28449111210032,
176.384962205932));
#13485=CARTESIAN_POINT('Ctrl Pts',(-55.9545655524391,-3.23079314429921,
176.725242297786));
#13486=CARTESIAN_POINT('Ctrl Pts',(-55.7610730366685,-3.12770940060629,
177.200137919422));
#13487=CARTESIAN_POINT('Ctrl Pts',(-55.6813772878146,-3.09105284269064,
177.349953976371));
#13488=CARTESIAN_POINT('Ctrl Pts',(-55.542047034587,-3.0325075684579,177.559861392858));
#13489=CARTESIAN_POINT('Ctrl Pts',(-55.4922962422521,-3.01237854056411,
177.627368088468));
#13490=CARTESIAN_POINT('Ctrl Pts',(-55.3864710916189,-2.97076694703694,
177.757099244203));
#13491=CARTESIAN_POINT('Ctrl Pts',(-55.3343400650611,-2.9517036220202,177.814670571915));
#13492=CARTESIAN_POINT('Ctrl Pts',(-55.2712257966423,-2.92704897744562,
177.878689530232));
#13493=CARTESIAN_POINT('Ctrl Pts',(-50.193114320713,-27.8005016688432,177.448440461337));
#13494=CARTESIAN_POINT('Ctrl Pts',(-50.1356777281885,-27.7780416249781,
177.514251363723));
#13495=CARTESIAN_POINT('Ctrl Pts',(-50.0768656935625,-27.751543311514,177.569181845458));
#13496=CARTESIAN_POINT('Ctrl Pts',(-49.9502510673185,-27.7006718917524,
177.678131488152));
#13497=CARTESIAN_POINT('Ctrl Pts',(-49.8836384545372,-27.6746069642733,
177.728584647058));
#13498=CARTESIAN_POINT('Ctrl Pts',(-49.6751767137455,-27.5945945456976,
177.866776279515));
#13499=CARTESIAN_POINT('Ctrl Pts',(-49.5241175159801,-27.5384622401806,
177.941191651987));
#13500=CARTESIAN_POINT('Ctrl Pts',(-49.052722448706,-27.3677108924734,178.102046365205));
#13501=CARTESIAN_POINT('Ctrl Pts',(-48.713006227557,-27.2491092781452,178.126053652285));
#13502=CARTESIAN_POINT('Ctrl Pts',(-47.7382795874562,-26.9019657740439,
177.942209528285));
#13503=CARTESIAN_POINT('Ctrl Pts',(-47.1597470877608,-26.6842880122364,
177.461567693823));
#13504=CARTESIAN_POINT('Ctrl Pts',(-46.658904710499,-26.3725604903201,176.179580952166));
#13505=CARTESIAN_POINT('Ctrl Pts',(-46.744016732095,-26.2835354545934,175.410971277798));
#13506=CARTESIAN_POINT('Ctrl Pts',(-47.5354179070377,-26.2224078706935,
174.242909311213));
#13507=CARTESIAN_POINT('Ctrl Pts',(-48.2245449656354,-26.2493771368743,
173.87343933243));
#13508=CARTESIAN_POINT('Ctrl Pts',(-49.6317089464608,-26.3060463238627,
173.871895146128));
#13509=CARTESIAN_POINT('Ctrl Pts',(-50.3230600395606,-26.332977077053,174.238655026377));
#13510=CARTESIAN_POINT('Ctrl Pts',(-51.1153496063116,-26.2743348509258,
175.387691644257));
#13511=CARTESIAN_POINT('Ctrl Pts',(-51.2096393582444,-26.1855070701005,
176.164686974611));
#13512=CARTESIAN_POINT('Ctrl Pts',(-50.7213268039385,-25.8775623946772,
177.442968877094));
#13513=CARTESIAN_POINT('Ctrl Pts',(-50.1473617008829,-25.6602454668112,
177.932812658479));
#13514=CARTESIAN_POINT('Ctrl Pts',(-48.8451246534299,-25.1962898596545,
178.190564242377));
#13515=CARTESIAN_POINT('Ctrl Pts',(-48.1356293396501,-24.9529458243571,
177.955714348281));
#13516=CARTESIAN_POINT('Ctrl Pts',(-47.2268076672755,-24.5631416907191,
176.954286183848));
#13517=CARTESIAN_POINT('Ctrl Pts',(-47.0395646158613,-24.4209960169422,
176.20954077848));
#13518=CARTESIAN_POINT('Ctrl Pts',(-47.370313215787,-24.2726666068476,174.855768290097));
#13519=CARTESIAN_POINT('Ctrl Pts',(-47.8845545017147,-24.265674947158,174.26583855031));
#13520=CARTESIAN_POINT('Ctrl Pts',(-49.1994460468846,-24.3046603227726,
173.764180115318));
#13521=CARTESIAN_POINT('Ctrl Pts',(-49.9762257647407,-24.3480555327739,
173.861039734223));
#13522=CARTESIAN_POINT('Ctrl Pts',(-51.1285193941288,-24.3574791486806,
174.66646218052));
#13523=CARTESIAN_POINT('Ctrl Pts',(-51.4882290443068,-24.3203491702665,
175.364132112564));
#13524=CARTESIAN_POINT('Ctrl Pts',(-51.4777341832408,-24.1036300286494,
176.755680066459));
#13525=CARTESIAN_POINT('Ctrl Pts',(-51.1141102527119,-23.9275319100486,
177.423612084264));
#13526=CARTESIAN_POINT('Ctrl Pts',(-49.9940329966114,-23.4994535030053,
178.148719290634));
#13527=CARTESIAN_POINT('Ctrl Pts',(-49.2531996565364,-23.2503850964097,
178.195074921104));
#13528=CARTESIAN_POINT('Ctrl Pts',(-48.0540724826088,-22.804580182732,177.607487959387));
#13529=CARTESIAN_POINT('Ctrl Pts',(-47.6174629086983,-22.6140260251447,
176.985139741962));
#13530=CARTESIAN_POINT('Ctrl Pts',(-47.4549919432363,-22.3698803060775,
175.609945370482));
#13531=CARTESIAN_POINT('Ctrl Pts',(-47.7329522193418,-22.3169255939418,
174.876470615888));
#13532=CARTESIAN_POINT('Ctrl Pts',(-48.8440385240951,-22.3059754149369,
173.902867041218));
#13533=CARTESIAN_POINT('Ctrl Pts',(-49.7035599970344,-22.3554674780819,
173.739637329099));
#13534=CARTESIAN_POINT('Ctrl Pts',(-51.1531706356154,-22.4011313967338,
174.265066374312));
#13535=CARTESIAN_POINT('Ctrl Pts',(-51.7115054154064,-22.3910761212842,
174.945624054023));
#13536=CARTESIAN_POINT('Ctrl Pts',(-51.9563259347572,-22.2045289991918,
176.459132103654));
#13537=CARTESIAN_POINT('Ctrl Pts',(-51.63765119649,-22.0251559400258,177.262331468575));
#13538=CARTESIAN_POINT('Ctrl Pts',(-50.4571461815608,-21.5627984935069,
178.149907937338));
#13539=CARTESIAN_POINT('Ctrl Pts',(-49.6222512854117,-21.2849471395443,
178.217719280236));
#13540=CARTESIAN_POINT('Ctrl Pts',(-48.3256452005116,-20.7988977065915,
177.525255091295));
#13541=CARTESIAN_POINT('Ctrl Pts',(-47.8935170509031,-20.5993012814682,
176.78942555283));
#13542=CARTESIAN_POINT('Ctrl Pts',(-47.9069259765589,-20.3679964193449,
175.264267840625));
#13543=CARTESIAN_POINT('Ctrl Pts',(-48.3565963500671,-20.33698501403,174.508050023486));
#13544=CARTESIAN_POINT('Ctrl Pts',(-49.7115395236169,-20.3645147337819,
173.767258025586));
#13545=CARTESIAN_POINT('Ctrl Pts',(-50.5919963646361,-20.4163759449694,
173.798730113887));
#13546=CARTESIAN_POINT('Ctrl Pts',(-51.8921615926268,-20.4324111199544,
174.637786957993));
#13547=CARTESIAN_POINT('Ctrl Pts',(-52.2870845316673,-20.391715494119,175.425932171935));
#13548=CARTESIAN_POINT('Ctrl Pts',(-52.1845249551972,-20.1359343420921,
176.949348485014));
#13549=CARTESIAN_POINT('Ctrl Pts',(-51.6978717551623,-19.9258306519252,
177.647217385389));
#13550=CARTESIAN_POINT('Ctrl Pts',(-50.3567743114224,-19.4332812849397,
178.229888643815));
#13551=CARTESIAN_POINT('Ctrl Pts',(-49.531482093434,-19.1564117811874,178.098575810452));
#13552=CARTESIAN_POINT('Ctrl Pts',(-48.4209526978951,-18.7085233315365,
177.123331466978));
#13553=CARTESIAN_POINT('Ctrl Pts',(-48.1597795720535,-18.5402167412103,
176.29718764283));
#13554=CARTESIAN_POINT('Ctrl Pts',(-48.5145782694716,-18.3739619700934,
174.800216258582));
#13555=CARTESIAN_POINT('Ctrl Pts',(-49.1216168980297,-18.3741927637648,
174.159897255644));
#13556=CARTESIAN_POINT('Ctrl Pts',(-50.6124880467131,-18.4256628314289,
173.74530968569));
#13557=CARTESIAN_POINT('Ctrl Pts',(-51.4570089590119,-18.472296203581,173.973986288395));
#13558=CARTESIAN_POINT('Ctrl Pts',(-52.5367755134872,-18.4465314340497,
175.076321400051));
#13559=CARTESIAN_POINT('Ctrl Pts',(-52.7461464663159,-18.3691716102472,
175.928004990245));
#13560=CARTESIAN_POINT('Ctrl Pts',(-52.3166330239091,-18.0526500335514,
177.376965544067));
#13561=CARTESIAN_POINT('Ctrl Pts',(-51.6857211698905,-17.8130496454,177.945754508989));
#13562=CARTESIAN_POINT('Ctrl Pts',(-50.2465394893753,-17.3007990625156,
178.194297846636));
#13563=CARTESIAN_POINT('Ctrl Pts',(-49.4703000985441,-17.0343670318334,
177.871754882023));
#13564=CARTESIAN_POINT('Ctrl Pts',(-48.6088763818932,-16.6321365971318,
176.648991214725));
#13565=CARTESIAN_POINT('Ctrl Pts',(-48.5409020769561,-16.5028432711256,
175.78526591443));
#13566=CARTESIAN_POINT('Ctrl Pts',(-49.2164515058916,-16.3991203888251,
174.401518908745));
#13567=CARTESIAN_POINT('Ctrl Pts',(-49.9496118192587,-16.4227354715302,
173.914202886417));
#13568=CARTESIAN_POINT('Ctrl Pts',(-51.4902606534728,-16.4861638259448,
173.836744887307));
#13569=CARTESIAN_POINT('Ctrl Pts',(-52.2697075969923,-16.5185243960147,
174.249627738192));
#13570=CARTESIAN_POINT('Ctrl Pts',(-53.0792623986938,-16.4399376212412,
175.566241461313));
#13571=CARTESIAN_POINT('Ctrl Pts',(-53.0958608617722,-16.3264383488088,
176.440260240546));
#13572=CARTESIAN_POINT('Ctrl Pts',(-52.3498924896565,-15.9464100326616,
177.743856795072));
#13573=CARTESIAN_POINT('Ctrl Pts',(-51.6136771994172,-15.6882407493956,
178.142477224647));
#13574=CARTESIAN_POINT('Ctrl Pts',(-50.1619939854693,-15.1743526813971,
178.045393567771));
#13575=CARTESIAN_POINT('Ctrl Pts',(-49.479535393056,-14.9249532161513,177.547481856475));
#13576=CARTESIAN_POINT('Ctrl Pts',(-48.9083003859244,-14.5811172796918,
176.154888290848));
#13577=CARTESIAN_POINT('Ctrl Pts',(-49.032687325759,-14.4872017268269,175.286386043965));
#13578=CARTESIAN_POINT('Ctrl Pts',(-50.002899927607,-14.4395306566209,174.08106638639));
#13579=CARTESIAN_POINT('Ctrl Pts',(-50.8258619899905,-14.4815667576624,
173.768688449528));
#13580=CARTESIAN_POINT('Ctrl Pts',(-52.3490472247602,-14.5391579602322,
174.044477097964));
#13581=CARTESIAN_POINT('Ctrl Pts',(-53.0108480437211,-14.5505369630929,
174.618897762295));
#13582=CARTESIAN_POINT('Ctrl Pts',(-53.508606726061,-14.41258118913,176.072854784516));
#13583=CARTESIAN_POINT('Ctrl Pts',(-53.3308496256547,-14.2605010523332,
176.92211652172));
#13584=CARTESIAN_POINT('Ctrl Pts',(-52.3234046589676,-13.8325238003689,
178.011250192421));
#13585=CARTESIAN_POINT('Ctrl Pts',(-51.5138129382755,-13.5585438056648,
178.229366209696));
#13586=CARTESIAN_POINT('Ctrl Pts',(-50.1182607249297,-13.0546721198729,
177.788098654291));
#13587=CARTESIAN_POINT('Ctrl Pts',(-49.5630188185408,-12.8308644828691,
177.140857971114));
#13588=CARTESIAN_POINT('Ctrl Pts',(-49.3219040202974,-12.5483689245281,
175.637957478437));
#13589=CARTESIAN_POINT('Ctrl Pts',(-49.6365594730894,-12.4926951709364,
174.821179942866));
#13590=CARTESIAN_POINT('Ctrl Pts',(-50.8450351424658,-12.4918253386163,
173.862170041067));
#13591=CARTESIAN_POINT('Ctrl Pts',(-51.7160671936879,-12.5420406725331,
173.742988789581));
#13592=CARTESIAN_POINT('Ctrl Pts',(-53.1380531234061,-12.5824907099911,
174.344563971126));
#13593=CARTESIAN_POINT('Ctrl Pts',(-53.661497991413,-12.565516429584,175.054752397452));
#13594=CARTESIAN_POINT('Ctrl Pts',(-53.8242077932451,-12.3622912981454,
176.579637740953));
#13595=CARTESIAN_POINT('Ctrl Pts',(-53.4635573374974,-12.1759538811977,
177.362604506387));
#13596=CARTESIAN_POINT('Ctrl Pts',(-52.2358756182636,-11.7031645393402,
178.179207046235));
#13597=CARTESIAN_POINT('Ctrl Pts',(-51.404471480006,-11.4266005921062,178.198059647233));
#13598=CARTESIAN_POINT('Ctrl Pts',(-50.1465877134854,-10.9499764840513,
177.440684540534));
#13599=CARTESIAN_POINT('Ctrl Pts',(-49.7512566691313,-10.7559713173261,
176.677961727673));
#13600=CARTESIAN_POINT('Ctrl Pts',(-49.8442980389787,-10.5402489724976,
175.152069846099));
#13601=CARTESIAN_POINT('Ctrl Pts',(-50.3336227209985,-10.5166703329192,
174.417963751365));
#13602=CARTESIAN_POINT('Ctrl Pts',(-51.729412313951,-10.5511670115394,173.750914008412));
#13603=CARTESIAN_POINT('Ctrl Pts',(-52.6055357660183,-10.6034581645062,
173.829125569603));
#13604=CARTESIAN_POINT('Ctrl Pts',(-53.8591972775733,-10.6090268187652,
174.739479897504));
#13605=CARTESIAN_POINT('Ctrl Pts',(-54.2075655427863,-10.559958422732,175.542285446703));
#13606=CARTESIAN_POINT('Ctrl Pts',(-54.0309723767407,-10.2919570312328,
177.05153449857));
#13607=CARTESIAN_POINT('Ctrl Pts',(-53.5065211660476,-10.0729835636969,
177.724885949439));
#13608=CARTESIAN_POINT('Ctrl Pts',(-52.1359327706082,-9.57501150980407,
178.231990439602));
#13609=CARTESIAN_POINT('Ctrl Pts',(-51.3168725161042,-9.29919601638729,
178.055337178134));
#13610=CARTESIAN_POINT('Ctrl Pts',(-50.258716477129,-8.86039345968628,177.014257444883));
#13611=CARTESIAN_POINT('Ctrl Pts',(-50.0419858596938,-8.70190296068798,
176.174822144773));
#13612=CARTESIAN_POINT('Ctrl Pts',(-50.4788136762356,-8.55014763089762,
174.697436550109));
#13613=CARTESIAN_POINT('Ctrl Pts',(-51.1165600370436,-8.55674976323144,
174.095019459488));
#13614=CARTESIAN_POINT('Ctrl Pts',(-52.6206590619166,-8.6128620697194,173.755704628284));
#13615=CARTESIAN_POINT('Ctrl Pts',(-53.456626592603,-8.65630954771657,174.029197443714));
#13616=CARTESIAN_POINT('Ctrl Pts',(-54.4781193003427,-8.6195332279715,175.187078119489));
#13617=CARTESIAN_POINT('Ctrl Pts',(-54.643602443466,-8.53353572012608,176.04949882023));
#13618=CARTESIAN_POINT('Ctrl Pts',(-54.1354947853707,-8.20096498746117,
177.472181687833));
#13619=CARTESIAN_POINT('Ctrl Pts',(-53.4760203027823,-7.95706608118669,
178.003825172765));
#13620=CARTESIAN_POINT('Ctrl Pts',(-52.0249165538012,-7.441132564782,178.167825277993));
#13621=CARTESIAN_POINT('Ctrl Pts',(-51.2723007652614,-7.17976116760829,
177.802466009854));
#13622=CARTESIAN_POINT('Ctrl Pts',(-50.4742318046734,-6.79179686888332,
176.539214575509));
#13623=CARTESIAN_POINT('Ctrl Pts',(-50.4508393849021,-6.66952799804251,
175.667365550039));
#13624=CARTESIAN_POINT('Ctrl Pts',(-51.1982775200671,-6.57992894303025,
174.318931761547));
#13625=CARTESIAN_POINT('Ctrl Pts',(-51.9567203354133,-6.60831910752051,
173.869388776842));
#13626=CARTESIAN_POINT('Ctrl Pts',(-53.5030461170827,-6.67180659392302,
173.876188814802));
#13627=CARTESIAN_POINT('Ctrl Pts',(-54.2579318048227,-6.70074853854407,
174.329266762268));
#13628=CARTESIAN_POINT('Ctrl Pts',(-54.9950541895712,-6.6067812144727,175.688231083653));
#13629=CARTESIAN_POINT('Ctrl Pts',(-54.9633937640365,-6.48434226598442,
176.556150922255));
#13630=CARTESIAN_POINT('Ctrl Pts',(-54.1573516980127,-6.0949735677162,177.812809342709));
#13631=CARTESIAN_POINT('Ctrl Pts',(-53.3979887985791,-5.83073710308303,
178.172806822259));
#13632=CARTESIAN_POINT('Ctrl Pts',(-51.9519097716579,-5.31810666795101,
177.994568269632));
#13633=CARTESIAN_POINT('Ctrl Pts',(-51.2952074816856,-5.0735953089356,177.458800517348));
#13634=CARTESIAN_POINT('Ctrl Pts',(-50.7993635736617,-4.74342220821161,
176.031468409862));
#13635=CARTESIAN_POINT('Ctrl Pts',(-50.9692613848378,-4.65940397939939,
175.170313217647));
#13636=CARTESIAN_POINT('Ctrl Pts',(-52.0040245669764,-4.62293999106357,
174.01934301833));
#13637=CARTESIAN_POINT('Ctrl Pts',(-52.8385688131003,-4.66759138415716,
173.754231358386));
#13638=CARTESIAN_POINT('Ctrl Pts',(-54.3414847379305,-4.72329909029368,
174.103969484305));
#13639=CARTESIAN_POINT('Ctrl Pts',(-54.9761466933045,-4.72791014175074,
174.714716972292));
#13640=CARTESIAN_POINT('Ctrl Pts',(-55.3975165431988,-4.57549651155636,
176.192173272167));
#13641=CARTESIAN_POINT('Ctrl Pts',(-55.1760506072609,-4.4148786220368,177.03103539143));
#13642=CARTESIAN_POINT('Ctrl Pts',(-54.1093043232961,-3.97451188101218,
178.061753391873));
#13643=CARTESIAN_POINT('Ctrl Pts',(-53.2902925544343,-3.69995792969149,
178.233822626392));
#13644=CARTESIAN_POINT('Ctrl Pts',(-51.9203920380846,-3.19963469730891,
177.711493690972));
#13645=CARTESIAN_POINT('Ctrl Pts',(-51.4044324721558,-2.98383265912278,
177.036002564632));
#13646=CARTESIAN_POINT('Ctrl Pts',(-51.237949425703,-2.71774512370317,175.525044339462));
#13647=CARTESIAN_POINT('Ctrl Pts',(-51.5957499271559,-2.66894330374766,
174.721509320474));
#13648=CARTESIAN_POINT('Ctrl Pts',(-52.8541051305037,-2.67783999801612,
173.825937213487));
#13649=CARTESIAN_POINT('Ctrl Pts',(-53.7315999697276,-2.7292086653859,173.7525048498));
#13650=CARTESIAN_POINT('Ctrl Pts',(-55.1208667949195,-2.76252327401043,
174.431246184642));
#13651=CARTESIAN_POINT('Ctrl Pts',(-55.6054709668258,-2.73893798071373,
175.167402226862));
#13652=CARTESIAN_POINT('Ctrl Pts',(-55.6603171863937,-2.58869274068622,
176.211840888345));
#13653=CARTESIAN_POINT('Ctrl Pts',(-55.6210463302226,-2.5392081864434,176.490448482462));
#13654=CARTESIAN_POINT('Ctrl Pts',(-55.4836397365907,-2.4479441182576,176.880586390838));
#13655=CARTESIAN_POINT('Ctrl Pts',(-55.4253285390117,-2.41535251334816,
177.005027857449));
#13656=CARTESIAN_POINT('Ctrl Pts',(-55.321414213033,-2.36345060131236,177.180440236558));
#13657=CARTESIAN_POINT('Ctrl Pts',(-55.2840225057543,-2.34563722905757,
177.23703696138));
#13658=CARTESIAN_POINT('Ctrl Pts',(-55.2039936793606,-2.30896761153951,
177.345998347345));
#13659=CARTESIAN_POINT('Ctrl Pts',(-55.1587206712145,-2.28906361698866,
177.401367187303));
#13660=CARTESIAN_POINT('Ctrl Pts',(-55.1161897096451,-2.27071607222657,
177.448351373365));
#13661=CARTESIAN_POINT('',(-49.6057233026533,-28.1882175989763,177.068114089093));
#13662=CARTESIAN_POINT('',(-50.193114320713,-27.8005016688432,177.448440461337));
#13663=CARTESIAN_POINT('Origin',(-49.8994188116831,-27.9943596339097,177.258277275215));
#13664=CARTESIAN_POINT('Ctrl Pts',(-49.6057233026533,-28.1882175989763,
177.068114089093));
#13665=CARTESIAN_POINT('Ctrl Pts',(-49.5663192275732,-28.1656109096198,
177.105925367078));
#13666=CARTESIAN_POINT('Ctrl Pts',(-49.5216854287654,-28.1457023853521,
177.148383027181));
#13667=CARTESIAN_POINT('Ctrl Pts',(-49.4301127133764,-28.1014695235449,
177.220446553382));
#13668=CARTESIAN_POINT('Ctrl Pts',(-49.3819809603125,-28.0788363277035,
177.253617740645));
#13669=CARTESIAN_POINT('Ctrl Pts',(-49.2321484222821,-28.0099337266433,
177.343479018307));
#13670=CARTESIAN_POINT('Ctrl Pts',(-49.1254026293825,-27.9629901656525,
177.390284377819));
#13671=CARTESIAN_POINT('Ctrl Pts',(-48.7929164986652,-27.8189908160803,
177.48590296908));
#13672=CARTESIAN_POINT('Ctrl Pts',(-48.55635218661,-27.7202377019268,177.490394220553));
#13673=CARTESIAN_POINT('Ctrl Pts',(-47.8840648999533,-27.4305281812212,
177.324447440169));
#13674=CARTESIAN_POINT('Ctrl Pts',(-47.5006474873523,-27.2497443022818,
176.963331771584));
#13675=CARTESIAN_POINT('Ctrl Pts',(-47.2040861213115,-26.9802047380462,
176.046394548579));
#13676=CARTESIAN_POINT('Ctrl Pts',(-47.2954018922066,-26.8917044501032,
175.506598760119));
#13677=CARTESIAN_POINT('Ctrl Pts',(-47.9062028356891,-26.7943163650827,
174.710326627486));
#13678=CARTESIAN_POINT('Ctrl Pts',(-48.4108882632775,-26.7850298620733,
174.47568647468));
#13679=CARTESIAN_POINT('Ctrl Pts',(-49.4081207961382,-26.7654318876047,
174.522051214009));
#13680=CARTESIAN_POINT('Ctrl Pts',(-49.8895805322777,-26.7512165827191,
174.803706734764));
#13681=CARTESIAN_POINT('Ctrl Pts',(-50.419859907048,-26.6406327974915,175.641132157405));
#13682=CARTESIAN_POINT('Ctrl Pts',(-50.4638072135826,-26.5414518590087,
176.190943138814));
#13683=CARTESIAN_POINT('Ctrl Pts',(-50.0902675056585,-26.258306693899,177.06820282525));
#13684=CARTESIAN_POINT('Ctrl Pts',(-49.6753169680471,-26.0710530131776,
177.393289133135));
#13685=CARTESIAN_POINT('Ctrl Pts',(-48.760110273011,-25.6803067135432,177.526354227003));
#13686=CARTESIAN_POINT('Ctrl Pts',(-48.2752065557733,-25.4795815288234,
177.333261554155));
#13687=CARTESIAN_POINT('Ctrl Pts',(-47.6834949732814,-25.1537104488559,
176.598820399841));
#13688=CARTESIAN_POINT('Ctrl Pts',(-47.581935800625,-25.0274199406948,176.066471856633));
#13689=CARTESIAN_POINT('Ctrl Pts',(-47.8743577335121,-24.8702793490883,
175.122570330099));
#13690=CARTESIAN_POINT('Ctrl Pts',(-48.2639300332364,-24.8386062285325,
174.72605490093));
#13691=CARTESIAN_POINT('Ctrl Pts',(-49.2134664973944,-24.8097944361078,
174.418869413643));
#13692=CARTESIAN_POINT('Ctrl Pts',(-49.7639560285487,-24.8089577046691,
174.513086690221));
#13693=CARTESIAN_POINT('Ctrl Pts',(-50.5601436025432,-24.7482854574026,
175.121296078095));
#13694=CARTESIAN_POINT('Ctrl Pts',(-50.7937850628585,-24.6861522884041,
175.625415363842));
#13695=CARTESIAN_POINT('Ctrl Pts',(-50.7513118113109,-24.4660502953853,
176.598470930813));
#13696=CARTESIAN_POINT('Ctrl Pts',(-50.4787452748198,-24.3068424850894,
177.056448064075));
#13697=CARTESIAN_POINT('Ctrl Pts',(-49.6755858463959,-23.9384579984121,
177.525629368769));
#13698=CARTESIAN_POINT('Ctrl Pts',(-49.1583261106009,-23.7318611386462,
177.529378707235));
#13699=CARTESIAN_POINT('Ctrl Pts',(-48.3492917504345,-23.3639427741862,
177.074636497803));
#13700=CARTESIAN_POINT('Ctrl Pts',(-48.0678997211374,-23.2027238239874,
176.620161976926));
#13701=CARTESIAN_POINT('Ctrl Pts',(-48.0133698591323,-22.9779683240005,
175.643265853549));
#13702=CARTESIAN_POINT('Ctrl Pts',(-48.2419634078688,-22.9148026311583,
175.13669620061));
#13703=CARTESIAN_POINT('Ctrl Pts',(-49.0648716087653,-22.8512007031896,
174.491772947554));
#13704=CARTESIAN_POINT('Ctrl Pts',(-49.6839608902416,-22.8528771386521,
174.405900021421));
#13705=CARTESIAN_POINT('Ctrl Pts',(-50.6991943315865,-22.8143164724711,
174.826217042058));
#13706=CARTESIAN_POINT('Ctrl Pts',(-51.0745700439279,-22.7701586995258,
175.322569579276));
#13707=CARTESIAN_POINT('Ctrl Pts',(-51.2073695092728,-22.5604456438022,
176.396956445951));
#13708=CARTESIAN_POINT('Ctrl Pts',(-50.9625278765238,-22.3963905325425,
176.94851178212));
#13709=CARTESIAN_POINT('Ctrl Pts',(-50.1139689940341,-21.9977514714476,
177.529315681618));
#13710=CARTESIAN_POINT('Ctrl Pts',(-49.5293219694751,-21.7666067892758,
177.544699935169));
#13711=CARTESIAN_POINT('Ctrl Pts',(-48.6567664449969,-21.3653910132907,
177.013098304479));
#13712=CARTESIAN_POINT('Ctrl Pts',(-48.383128531039,-21.1949054338945,176.477577858981));
#13713=CARTESIAN_POINT('Ctrl Pts',(-48.4582777380059,-20.975048733324,175.402873064259));
#13714=CARTESIAN_POINT('Ctrl Pts',(-48.8055781932514,-20.9254744005303,
174.886960050279));
#13715=CARTESIAN_POINT('Ctrl Pts',(-49.7998797569528,-20.8818943796597,
174.412232108109));
#13716=CARTESIAN_POINT('Ctrl Pts',(-50.4230224397188,-20.885216808613,174.464849386198));
#13717=CARTESIAN_POINT('Ctrl Pts',(-51.3220781362712,-20.8236066704411,
175.100442044691));
#13718=CARTESIAN_POINT('Ctrl Pts',(-51.5785314568021,-20.7546592125729,
175.670463366294));
#13719=CARTESIAN_POINT('Ctrl Pts',(-51.4682882413066,-20.5004564781585,
176.732562819156));
#13720=CARTESIAN_POINT('Ctrl Pts',(-51.1076577914431,-20.313201754554,177.207532153307));
#13721=CARTESIAN_POINT('Ctrl Pts',(-50.156411198824,-19.8953744930702,177.56803029022));
#13722=CARTESIAN_POINT('Ctrl Pts',(-49.5878400685962,-19.6691878319784,
177.446385146947));
#13723=CARTESIAN_POINT('Ctrl Pts',(-48.852079415717,-19.2920053425884,176.716949064536));
#13724=CARTESIAN_POINT('Ctrl Pts',(-48.7034574890464,-19.1464856081966,
176.127114392609));
#13725=CARTESIAN_POINT('Ctrl Pts',(-49.017896392823,-18.9721498737463,175.084671234462));
#13726=CARTESIAN_POINT('Ctrl Pts',(-49.4761175027563,-18.9421345006494,
174.655217811997));
#13727=CARTESIAN_POINT('Ctrl Pts',(-50.5469446991098,-18.915664221674,174.415005106013));
#13728=CARTESIAN_POINT('Ctrl Pts',(-51.1421889783774,-18.9127734302845,
174.605352538579));
#13729=CARTESIAN_POINT('Ctrl Pts',(-51.8771202801842,-18.8200557591642,
175.418505113175));
#13730=CARTESIAN_POINT('Ctrl Pts',(-52.0018165496213,-18.7275436462981,
176.022835099282));
#13731=CARTESIAN_POINT('Ctrl Pts',(-51.6614363875286,-18.4266465795959,
177.027259608014));
#13732=CARTESIAN_POINT('Ctrl Pts',(-51.2055166082591,-18.2218754080822,
177.403206831321));
#13733=CARTESIAN_POINT('Ctrl Pts',(-50.1969770591628,-17.7923688711786,
177.524973109627));
#13734=CARTESIAN_POINT('Ctrl Pts',(-49.6679526067506,-17.5720619524455,
177.267256975221));
#13735=CARTESIAN_POINT('Ctrl Pts',(-49.1179984398299,-17.2329564925234,
176.379271882249));
#13736=CARTESIAN_POINT('Ctrl Pts',(-49.1058293111544,-17.1129691055462,
175.766207634738));
#13737=CARTESIAN_POINT('Ctrl Pts',(-49.6421979468107,-16.981953011196,174.814805282058));
#13738=CARTESIAN_POINT('Ctrl Pts',(-50.1794692968359,-16.96896833752,174.497498655776));
#13739=CARTESIAN_POINT('Ctrl Pts',(-51.2815033366288,-16.9462509137644,
174.497183387712));
#13740=CARTESIAN_POINT('Ctrl Pts',(-51.8206810039433,-16.9333636766774,
174.813868002799));
#13741=CARTESIAN_POINT('Ctrl Pts',(-52.3579329121243,-16.8019633847227,
175.767995550527));
#13742=CARTESIAN_POINT('Ctrl Pts',(-52.3444015552563,-16.6811074119364,
176.384253300385));
#13743=CARTESIAN_POINT('Ctrl Pts',(-51.7908025496479,-16.3412377353734,
177.270036214878));
#13744=CARTESIAN_POINT('Ctrl Pts',(-51.2640575414935,-16.1220052064028,
177.524939199898));
#13745=CARTESIAN_POINT('Ctrl Pts',(-50.2584821099884,-15.6936926334193,
177.402964762685));
#13746=CARTESIAN_POINT('Ctrl Pts',(-49.8024659570259,-15.4891340123335,
177.028965203342));
#13747=CARTESIAN_POINT('Ctrl Pts',(-49.4615190985809,-15.1881425443655,
176.024838210267));
#13748=CARTESIAN_POINT('Ctrl Pts',(-49.584917871472,-15.0951235636284,175.418993178211));
#13749=CARTESIAN_POINT('Ctrl Pts',(-50.3224323861862,-15.0022736039987,
174.603877612758));
#13750=CARTESIAN_POINT('Ctrl Pts',(-50.9209588419739,-14.9994851008446,
174.413907495741));
#13751=CARTESIAN_POINT('Ctrl Pts',(-51.9913299824675,-14.9728180278691,
174.658436700836));
#13752=CARTESIAN_POINT('Ctrl Pts',(-52.4458562262816,-14.942768055369,175.086526075902));
#13753=CARTESIAN_POINT('Ctrl Pts',(-52.7589234637054,-14.768747576336,176.126312497655));
#13754=CARTESIAN_POINT('Ctrl Pts',(-52.6119738826496,-14.6237809758753,
176.715478760326));
#13755=CARTESIAN_POINT('Ctrl Pts',(-51.8767097042875,-14.2467264136774,
177.445252299972));
#13756=CARTESIAN_POINT('Ctrl Pts',(-51.3074205647036,-14.0201741438431,
177.568755188896));
#13757=CARTESIAN_POINT('Ctrl Pts',(-50.3534291722187,-13.6011459302421,
177.20657523661));
#13758=CARTESIAN_POINT('Ctrl Pts',(-49.9921349812078,-13.4131957453291,
176.728222347554));
#13759=CARTESIAN_POINT('Ctrl Pts',(-49.8860852889645,-13.159806046502,175.66552302478));
#13760=CARTESIAN_POINT('Ctrl Pts',(-50.1425376823364,-13.0914495220188,
175.099033652958));
#13761=CARTESIAN_POINT('Ctrl Pts',(-51.0393482876635,-13.0300320803285,
174.465742160163));
#13762=CARTESIAN_POINT('Ctrl Pts',(-51.661049564308,-13.0333384108268,174.411629490546));
#13763=CARTESIAN_POINT('Ctrl Pts',(-52.6556849728402,-12.9898139344045,
174.885756683857));
#13764=CARTESIAN_POINT('Ctrl Pts',(-53.0050117718212,-12.9403514819039,
175.401975295897));
#13765=CARTESIAN_POINT('Ctrl Pts',(-53.0797917942593,-12.7198628954119,
176.47950485369));
#13766=CARTESIAN_POINT('Ctrl Pts',(-52.8035180796908,-12.5482535501767,
177.017249165378));
#13767=CARTESIAN_POINT('Ctrl Pts',(-51.928756778869,-12.1465816152287,177.545168184464));
#13768=CARTESIAN_POINT('Ctrl Pts',(-51.3476399628683,-11.9168238447545,
177.52855345072));
#13769=CARTESIAN_POINT('Ctrl Pts',(-50.5013329357435,-11.5191203268418,
176.948730973903));
#13770=CARTESIAN_POINT('Ctrl Pts',(-50.2557375091139,-11.3551615877155,
176.398843509589));
#13771=CARTESIAN_POINT('Ctrl Pts',(-50.3877927376681,-11.145398461788,175.324825412843));
#13772=CARTESIAN_POINT('Ctrl Pts',(-50.762684868614,-11.1008426423184,174.826271833705));
#13773=CARTESIAN_POINT('Ctrl Pts',(-51.7811268292925,-11.0622619854364,
174.405264562934));
#13774=CARTESIAN_POINT('Ctrl Pts',(-52.4028793467296,-11.063958202758,174.492793292778));
#13775=CARTESIAN_POINT('Ctrl Pts',(-53.2632154661256,-10.9967409315864,
175.172494096186));
#13776=CARTESIAN_POINT('Ctrl Pts',(-53.4886849878534,-10.9225114509841,
175.750866168407));
#13777=CARTESIAN_POINT('Ctrl Pts',(-53.3251423960266,-10.6565821386363,
176.805379202472));
#13778=CARTESIAN_POINT('Ctrl Pts',(-52.9407422532226,-10.465785944074,177.259010843821));
#13779=CARTESIAN_POINT('Ctrl Pts',(-51.9697953271392,-10.0433159226031,
177.565260787091));
#13780=CARTESIAN_POINT('Ctrl Pts',(-51.4073968434514,-9.81808614025534,
177.411394538556));
#13781=CARTESIAN_POINT('Ctrl Pts',(-50.7116066211125,-9.44884954788431,
176.639139203566));
#13782=CARTESIAN_POINT('Ctrl Pts',(-50.5960828064805,-9.30833579234248,
176.038056438509));
#13783=CARTESIAN_POINT('Ctrl Pts',(-50.9640903737478,-9.14636922546571,
175.0167568496));
#13784=CARTESIAN_POINT('Ctrl Pts',(-51.4414488535671,-9.12058052193367,
174.612974652851));
#13785=CARTESIAN_POINT('Ctrl Pts',(-52.5249204417031,-9.09513784416194,
174.426509843431));
#13786=CARTESIAN_POINT('Ctrl Pts',(-53.1088418277628,-9.09114996369398,
174.646804488947));
#13787=CARTESIAN_POINT('Ctrl Pts',(-53.801661971168,-8.98942785386125,175.498626413927));
#13788=CARTESIAN_POINT('Ctrl Pts',(-53.8945655335682,-8.89052591977855,
176.108945227942));
#13789=CARTESIAN_POINT('Ctrl Pts',(-53.5007325042087,-8.57967938234873,
177.090495387502));
#13790=CARTESIAN_POINT('Ctrl Pts',(-53.0228734977247,-8.36926263084827,
177.439659990072));
#13791=CARTESIAN_POINT('Ctrl Pts',(-52.0134388460396,-7.941561484533,177.502665384752));
#13792=CARTESIAN_POINT('Ctrl Pts',(-51.5009539686643,-7.72503451842822,
177.217498325365));
#13793=CARTESIAN_POINT('Ctrl Pts',(-50.9958226444158,-7.39311721565184,
176.298072843289));
#13794=CARTESIAN_POINT('Ctrl Pts',(-51.0149583411939,-7.28021855779389,
175.684524900703));
#13795=CARTESIAN_POINT('Ctrl Pts',(-51.602189663565,-7.15816051285745,174.759352960774));
#13796=CARTESIAN_POINT('Ctrl Pts',(-52.1561751142271,-7.14821693453925,
174.470064567704));
#13797=CARTESIAN_POINT('Ctrl Pts',(-53.257284967077,-7.12553378294388,174.528734890764));
#13798=CARTESIAN_POINT('Ctrl Pts',(-53.7798318899166,-7.10813319884164,
174.876062446534));
#13799=CARTESIAN_POINT('Ctrl Pts',(-54.263309402104,-6.96831483361839,175.852098283111));
#13800=CARTESIAN_POINT('Ctrl Pts',(-54.2182177005742,-6.84182185515181,
176.463118413));
#13801=CARTESIAN_POINT('Ctrl Pts',(-53.620326169719,-6.49215310837908,177.317242942806));
#13802=CARTESIAN_POINT('Ctrl Pts',(-53.0815432796407,-6.27162057701451,
177.542753252723));
#13803=CARTESIAN_POINT('Ctrl Pts',(-52.0813405764902,-5.84340716815714,
177.363069610828));
#13804=CARTESIAN_POINT('Ctrl Pts',(-51.6451899827477,-5.64252013198273,
176.962963727015));
#13805=CARTESIAN_POINT('Ctrl Pts',(-51.3585173428123,-5.35236886702559,
175.939011043839));
#13806=CARTESIAN_POINT('Ctrl Pts',(-51.5164782073777,-5.2645103327986,175.337256223397));
#13807=CARTESIAN_POINT('Ctrl Pts',(-52.2924300679745,-5.18119763163266,
174.565366155634));
#13808=CARTESIAN_POINT('Ctrl Pts',(-52.8973452213176,-5.1801045826173,174.406680096152));
#13809=CARTESIAN_POINT('Ctrl Pts',(-53.956162505713,-5.14973256956073,174.705214074754));
#13810=CARTESIAN_POINT('Ctrl Pts',(-54.3874707400874,-5.11629663400306,
175.155234787811));
#13811=CARTESIAN_POINT('Ctrl Pts',(-54.6460006492434,-4.93091655090319,
176.210608238885));
#13812=CARTESIAN_POINT('Ctrl Pts',(-54.4681690759566,-4.77980797892323,
176.790635503925));
#13813=CARTESIAN_POINT('Ctrl Pts',(-53.6946945331643,-4.3956772156615,177.47627897342));
#13814=CARTESIAN_POINT('Ctrl Pts',(-53.1174419759953,-4.16620647621949,
177.565792133827));
#13815=CARTESIAN_POINT('Ctrl Pts',(-52.1878574222778,-3.75385530866336,
177.150829002666));
#13816=CARTESIAN_POINT('Ctrl Pts',(-51.8529856411974,-3.5715083216093,176.654958973924));
#13817=CARTESIAN_POINT('Ctrl Pts',(-51.8010050251376,-3.32706416715232,
175.583828138226));
#13818=CARTESIAN_POINT('Ctrl Pts',(-52.0854219579878,-3.26527816982496,
175.031488604324));
#13819=CARTESIAN_POINT('Ctrl Pts',(-53.0170398348192,-3.20959915076688,
174.444132662069));
#13820=CARTESIAN_POINT('Ctrl Pts',(-53.6416591927321,-3.21325709639781,
174.423035709656));
#13821=CARTESIAN_POINT('Ctrl Pts',(-54.6090153740635,-3.16498595686182,
174.948967905512));
#13822=CARTESIAN_POINT('Ctrl Pts',(-54.9308286711417,-3.10893139642228,
175.48555871107));
#13823=CARTESIAN_POINT('Ctrl Pts',(-54.9426665516143,-2.95192631073098,
176.218540695264));
#13824=CARTESIAN_POINT('Ctrl Pts',(-54.9070365263685,-2.90171640292054,
176.413787336324));
#13825=CARTESIAN_POINT('Ctrl Pts',(-54.8013987998623,-2.81782847468563,
176.681821034794));
#13826=CARTESIAN_POINT('Ctrl Pts',(-54.7570848510793,-2.78787367953458,
176.767627228561));
#13827=CARTESIAN_POINT('Ctrl Pts',(-54.6793253219128,-2.74078668455889,
176.887592985838));
#13828=CARTESIAN_POINT('Ctrl Pts',(-54.651529701944,-2.72473899696222,176.926133356148));
#13829=CARTESIAN_POINT('Ctrl Pts',(-54.5925997439423,-2.69209575899625,
176.999824075839));
#13830=CARTESIAN_POINT('Ctrl Pts',(-54.5641015373143,-2.67654794454284,
177.031971691023));
#13831=CARTESIAN_POINT('Ctrl Pts',(-54.5288628436534,-2.65870383148502,
177.068203177065));
#13832=CARTESIAN_POINT('Ctrl Pts',(-50.193114320713,-27.8005016688432,177.448440461337));
#13833=CARTESIAN_POINT('Ctrl Pts',(-50.1356777281885,-27.7780416249781,
177.514251363723));
#13834=CARTESIAN_POINT('Ctrl Pts',(-50.0768656935625,-27.751543311514,177.569181845458));
#13835=CARTESIAN_POINT('Ctrl Pts',(-49.9502510673185,-27.7006718917524,
177.678131488152));
#13836=CARTESIAN_POINT('Ctrl Pts',(-49.8836384545372,-27.6746069642733,
177.728584647058));
#13837=CARTESIAN_POINT('Ctrl Pts',(-49.6751767137455,-27.5945945456976,
177.866776279515));
#13838=CARTESIAN_POINT('Ctrl Pts',(-49.5241175159801,-27.5384622401806,
177.941191651987));
#13839=CARTESIAN_POINT('Ctrl Pts',(-49.052722448706,-27.3677108924734,178.102046365205));
#13840=CARTESIAN_POINT('Ctrl Pts',(-48.713006227557,-27.2491092781452,178.126053652285));
#13841=CARTESIAN_POINT('Ctrl Pts',(-47.7382795874562,-26.9019657740439,
177.942209528285));
#13842=CARTESIAN_POINT('Ctrl Pts',(-47.1597470877608,-26.6842880122364,
177.461567693823));
#13843=CARTESIAN_POINT('Ctrl Pts',(-46.658904710499,-26.3725604903201,176.179580952166));
#13844=CARTESIAN_POINT('Ctrl Pts',(-46.744016732095,-26.2835354545934,175.410971277798));
#13845=CARTESIAN_POINT('Ctrl Pts',(-47.5354179070377,-26.2224078706935,
174.242909311213));
#13846=CARTESIAN_POINT('Ctrl Pts',(-48.2245449656354,-26.2493771368743,
173.87343933243));
#13847=CARTESIAN_POINT('Ctrl Pts',(-49.6317089464608,-26.3060463238627,
173.871895146128));
#13848=CARTESIAN_POINT('Ctrl Pts',(-50.3230600395606,-26.332977077053,174.238655026377));
#13849=CARTESIAN_POINT('Ctrl Pts',(-51.1153496063116,-26.2743348509258,
175.387691644257));
#13850=CARTESIAN_POINT('Ctrl Pts',(-51.2096393582444,-26.1855070701005,
176.164686974611));
#13851=CARTESIAN_POINT('Ctrl Pts',(-50.7213268039385,-25.8775623946772,
177.442968877094));
#13852=CARTESIAN_POINT('Ctrl Pts',(-50.1473617008829,-25.6602454668112,
177.932812658479));
#13853=CARTESIAN_POINT('Ctrl Pts',(-48.8451246534299,-25.1962898596545,
178.190564242377));
#13854=CARTESIAN_POINT('Ctrl Pts',(-48.1356293396501,-24.9529458243571,
177.955714348281));
#13855=CARTESIAN_POINT('Ctrl Pts',(-47.2268076672755,-24.5631416907191,
176.954286183848));
#13856=CARTESIAN_POINT('Ctrl Pts',(-47.0395646158613,-24.4209960169422,
176.20954077848));
#13857=CARTESIAN_POINT('Ctrl Pts',(-47.370313215787,-24.2726666068476,174.855768290097));
#13858=CARTESIAN_POINT('Ctrl Pts',(-47.8845545017147,-24.265674947158,174.26583855031));
#13859=CARTESIAN_POINT('Ctrl Pts',(-49.1994460468846,-24.3046603227726,
173.764180115318));
#13860=CARTESIAN_POINT('Ctrl Pts',(-49.9762257647407,-24.3480555327739,
173.861039734223));
#13861=CARTESIAN_POINT('Ctrl Pts',(-51.1285193941288,-24.3574791486806,
174.66646218052));
#13862=CARTESIAN_POINT('Ctrl Pts',(-51.4882290443068,-24.3203491702665,
175.364132112564));
#13863=CARTESIAN_POINT('Ctrl Pts',(-51.4777341832408,-24.1036300286494,
176.755680066459));
#13864=CARTESIAN_POINT('Ctrl Pts',(-51.1141102527119,-23.9275319100486,
177.423612084264));
#13865=CARTESIAN_POINT('Ctrl Pts',(-49.9940329966114,-23.4994535030053,
178.148719290634));
#13866=CARTESIAN_POINT('Ctrl Pts',(-49.2531996565364,-23.2503850964097,
178.195074921104));
#13867=CARTESIAN_POINT('Ctrl Pts',(-48.0540724826088,-22.804580182732,177.607487959387));
#13868=CARTESIAN_POINT('Ctrl Pts',(-47.6174629086983,-22.6140260251447,
176.985139741962));
#13869=CARTESIAN_POINT('Ctrl Pts',(-47.4549919432363,-22.3698803060775,
175.609945370482));
#13870=CARTESIAN_POINT('Ctrl Pts',(-47.7329522193418,-22.3169255939418,
174.876470615888));
#13871=CARTESIAN_POINT('Ctrl Pts',(-48.8440385240951,-22.3059754149369,
173.902867041218));
#13872=CARTESIAN_POINT('Ctrl Pts',(-49.7035599970344,-22.3554674780819,
173.739637329099));
#13873=CARTESIAN_POINT('Ctrl Pts',(-51.1531706356154,-22.4011313967338,
174.265066374312));
#13874=CARTESIAN_POINT('Ctrl Pts',(-51.7115054154064,-22.3910761212842,
174.945624054023));
#13875=CARTESIAN_POINT('Ctrl Pts',(-51.9563259347572,-22.2045289991918,
176.459132103654));
#13876=CARTESIAN_POINT('Ctrl Pts',(-51.63765119649,-22.0251559400258,177.262331468575));
#13877=CARTESIAN_POINT('Ctrl Pts',(-50.4571461815608,-21.5627984935069,
178.149907937338));
#13878=CARTESIAN_POINT('Ctrl Pts',(-49.6222512854117,-21.2849471395443,
178.217719280236));
#13879=CARTESIAN_POINT('Ctrl Pts',(-48.3256452005116,-20.7988977065915,
177.525255091295));
#13880=CARTESIAN_POINT('Ctrl Pts',(-47.8935170509031,-20.5993012814682,
176.78942555283));
#13881=CARTESIAN_POINT('Ctrl Pts',(-47.9069259765589,-20.3679964193449,
175.264267840625));
#13882=CARTESIAN_POINT('Ctrl Pts',(-48.3565963500671,-20.33698501403,174.508050023486));
#13883=CARTESIAN_POINT('Ctrl Pts',(-49.7115395236169,-20.3645147337819,
173.767258025586));
#13884=CARTESIAN_POINT('Ctrl Pts',(-50.5919963646361,-20.4163759449694,
173.798730113887));
#13885=CARTESIAN_POINT('Ctrl Pts',(-51.8921615926268,-20.4324111199544,
174.637786957993));
#13886=CARTESIAN_POINT('Ctrl Pts',(-52.2870845316673,-20.391715494119,175.425932171935));
#13887=CARTESIAN_POINT('Ctrl Pts',(-52.1845249551972,-20.1359343420921,
176.949348485014));
#13888=CARTESIAN_POINT('Ctrl Pts',(-51.6978717551623,-19.9258306519252,
177.647217385389));
#13889=CARTESIAN_POINT('Ctrl Pts',(-50.3567743114224,-19.4332812849397,
178.229888643815));
#13890=CARTESIAN_POINT('Ctrl Pts',(-49.531482093434,-19.1564117811874,178.098575810452));
#13891=CARTESIAN_POINT('Ctrl Pts',(-48.4209526978951,-18.7085233315365,
177.123331466978));
#13892=CARTESIAN_POINT('Ctrl Pts',(-48.1597795720535,-18.5402167412103,
176.29718764283));
#13893=CARTESIAN_POINT('Ctrl Pts',(-48.5145782694716,-18.3739619700934,
174.800216258582));
#13894=CARTESIAN_POINT('Ctrl Pts',(-49.1216168980297,-18.3741927637648,
174.159897255644));
#13895=CARTESIAN_POINT('Ctrl Pts',(-50.6124880467131,-18.4256628314289,
173.74530968569));
#13896=CARTESIAN_POINT('Ctrl Pts',(-51.4570089590119,-18.472296203581,173.973986288395));
#13897=CARTESIAN_POINT('Ctrl Pts',(-52.5367755134872,-18.4465314340497,
175.076321400051));
#13898=CARTESIAN_POINT('Ctrl Pts',(-52.7461464663159,-18.3691716102472,
175.928004990245));
#13899=CARTESIAN_POINT('Ctrl Pts',(-52.3166330239091,-18.0526500335514,
177.376965544067));
#13900=CARTESIAN_POINT('Ctrl Pts',(-51.6857211698905,-17.8130496454,177.945754508989));
#13901=CARTESIAN_POINT('Ctrl Pts',(-50.2465394893753,-17.3007990625156,
178.194297846636));
#13902=CARTESIAN_POINT('Ctrl Pts',(-49.4703000985441,-17.0343670318334,
177.871754882023));
#13903=CARTESIAN_POINT('Ctrl Pts',(-48.6088763818932,-16.6321365971318,
176.648991214725));
#13904=CARTESIAN_POINT('Ctrl Pts',(-48.5409020769561,-16.5028432711256,
175.78526591443));
#13905=CARTESIAN_POINT('Ctrl Pts',(-49.2164515058916,-16.3991203888251,
174.401518908745));
#13906=CARTESIAN_POINT('Ctrl Pts',(-49.9496118192587,-16.4227354715302,
173.914202886417));
#13907=CARTESIAN_POINT('Ctrl Pts',(-51.4902606534728,-16.4861638259448,
173.836744887307));
#13908=CARTESIAN_POINT('Ctrl Pts',(-52.2697075969923,-16.5185243960147,
174.249627738192));
#13909=CARTESIAN_POINT('Ctrl Pts',(-53.0792623986938,-16.4399376212412,
175.566241461313));
#13910=CARTESIAN_POINT('Ctrl Pts',(-53.0958608617722,-16.3264383488088,
176.440260240546));
#13911=CARTESIAN_POINT('Ctrl Pts',(-52.3498924896565,-15.9464100326616,
177.743856795072));
#13912=CARTESIAN_POINT('Ctrl Pts',(-51.6136771994172,-15.6882407493956,
178.142477224647));
#13913=CARTESIAN_POINT('Ctrl Pts',(-50.1619939854693,-15.1743526813971,
178.045393567771));
#13914=CARTESIAN_POINT('Ctrl Pts',(-49.479535393056,-14.9249532161513,177.547481856475));
#13915=CARTESIAN_POINT('Ctrl Pts',(-48.9083003859244,-14.5811172796918,
176.154888290848));
#13916=CARTESIAN_POINT('Ctrl Pts',(-49.032687325759,-14.4872017268269,175.286386043965));
#13917=CARTESIAN_POINT('Ctrl Pts',(-50.002899927607,-14.4395306566209,174.08106638639));
#13918=CARTESIAN_POINT('Ctrl Pts',(-50.8258619899905,-14.4815667576624,
173.768688449528));
#13919=CARTESIAN_POINT('Ctrl Pts',(-52.3490472247602,-14.5391579602322,
174.044477097964));
#13920=CARTESIAN_POINT('Ctrl Pts',(-53.0108480437211,-14.5505369630929,
174.618897762295));
#13921=CARTESIAN_POINT('Ctrl Pts',(-53.508606726061,-14.41258118913,176.072854784516));
#13922=CARTESIAN_POINT('Ctrl Pts',(-53.3308496256547,-14.2605010523332,
176.92211652172));
#13923=CARTESIAN_POINT('Ctrl Pts',(-52.3234046589676,-13.8325238003689,
178.011250192421));
#13924=CARTESIAN_POINT('Ctrl Pts',(-51.5138129382755,-13.5585438056648,
178.229366209696));
#13925=CARTESIAN_POINT('Ctrl Pts',(-50.1182607249297,-13.0546721198729,
177.788098654291));
#13926=CARTESIAN_POINT('Ctrl Pts',(-49.5630188185408,-12.8308644828691,
177.140857971114));
#13927=CARTESIAN_POINT('Ctrl Pts',(-49.3219040202974,-12.5483689245281,
175.637957478437));
#13928=CARTESIAN_POINT('Ctrl Pts',(-49.6365594730894,-12.4926951709364,
174.821179942866));
#13929=CARTESIAN_POINT('Ctrl Pts',(-50.8450351424658,-12.4918253386163,
173.862170041067));
#13930=CARTESIAN_POINT('Ctrl Pts',(-51.7160671936879,-12.5420406725331,
173.742988789581));
#13931=CARTESIAN_POINT('Ctrl Pts',(-53.1380531234061,-12.5824907099911,
174.344563971126));
#13932=CARTESIAN_POINT('Ctrl Pts',(-53.661497991413,-12.565516429584,175.054752397452));
#13933=CARTESIAN_POINT('Ctrl Pts',(-53.8242077932451,-12.3622912981454,
176.579637740953));
#13934=CARTESIAN_POINT('Ctrl Pts',(-53.4635573374974,-12.1759538811977,
177.362604506387));
#13935=CARTESIAN_POINT('Ctrl Pts',(-52.2358756182636,-11.7031645393402,
178.179207046235));
#13936=CARTESIAN_POINT('Ctrl Pts',(-51.404471480006,-11.4266005921062,178.198059647233));
#13937=CARTESIAN_POINT('Ctrl Pts',(-50.1465877134854,-10.9499764840513,
177.440684540534));
#13938=CARTESIAN_POINT('Ctrl Pts',(-49.7512566691313,-10.7559713173261,
176.677961727673));
#13939=CARTESIAN_POINT('Ctrl Pts',(-49.8442980389787,-10.5402489724976,
175.152069846099));
#13940=CARTESIAN_POINT('Ctrl Pts',(-50.3336227209985,-10.5166703329192,
174.417963751365));
#13941=CARTESIAN_POINT('Ctrl Pts',(-51.729412313951,-10.5511670115394,173.750914008412));
#13942=CARTESIAN_POINT('Ctrl Pts',(-52.6055357660183,-10.6034581645062,
173.829125569603));
#13943=CARTESIAN_POINT('Ctrl Pts',(-53.8591972775733,-10.6090268187652,
174.739479897504));
#13944=CARTESIAN_POINT('Ctrl Pts',(-54.2075655427863,-10.559958422732,175.542285446703));
#13945=CARTESIAN_POINT('Ctrl Pts',(-54.0309723767407,-10.2919570312328,
177.05153449857));
#13946=CARTESIAN_POINT('Ctrl Pts',(-53.5065211660476,-10.0729835636969,
177.724885949439));
#13947=CARTESIAN_POINT('Ctrl Pts',(-52.1359327706082,-9.57501150980407,
178.231990439602));
#13948=CARTESIAN_POINT('Ctrl Pts',(-51.3168725161042,-9.29919601638729,
178.055337178134));
#13949=CARTESIAN_POINT('Ctrl Pts',(-50.258716477129,-8.86039345968628,177.014257444883));
#13950=CARTESIAN_POINT('Ctrl Pts',(-50.0419858596938,-8.70190296068798,
176.174822144773));
#13951=CARTESIAN_POINT('Ctrl Pts',(-50.4788136762356,-8.55014763089762,
174.697436550109));
#13952=CARTESIAN_POINT('Ctrl Pts',(-51.1165600370436,-8.55674976323144,
174.095019459488));
#13953=CARTESIAN_POINT('Ctrl Pts',(-52.6206590619166,-8.6128620697194,173.755704628284));
#13954=CARTESIAN_POINT('Ctrl Pts',(-53.456626592603,-8.65630954771657,174.029197443714));
#13955=CARTESIAN_POINT('Ctrl Pts',(-54.4781193003427,-8.6195332279715,175.187078119489));
#13956=CARTESIAN_POINT('Ctrl Pts',(-54.643602443466,-8.53353572012608,176.04949882023));
#13957=CARTESIAN_POINT('Ctrl Pts',(-54.1354947853707,-8.20096498746117,
177.472181687833));
#13958=CARTESIAN_POINT('Ctrl Pts',(-53.4760203027823,-7.95706608118669,
178.003825172765));
#13959=CARTESIAN_POINT('Ctrl Pts',(-52.0249165538012,-7.441132564782,178.167825277993));
#13960=CARTESIAN_POINT('Ctrl Pts',(-51.2723007652614,-7.17976116760829,
177.802466009854));
#13961=CARTESIAN_POINT('Ctrl Pts',(-50.4742318046734,-6.79179686888332,
176.539214575509));
#13962=CARTESIAN_POINT('Ctrl Pts',(-50.4508393849021,-6.66952799804251,
175.667365550039));
#13963=CARTESIAN_POINT('Ctrl Pts',(-51.1982775200671,-6.57992894303025,
174.318931761547));
#13964=CARTESIAN_POINT('Ctrl Pts',(-51.9567203354133,-6.60831910752051,
173.869388776842));
#13965=CARTESIAN_POINT('Ctrl Pts',(-53.5030461170827,-6.67180659392302,
173.876188814802));
#13966=CARTESIAN_POINT('Ctrl Pts',(-54.2579318048227,-6.70074853854407,
174.329266762268));
#13967=CARTESIAN_POINT('Ctrl Pts',(-54.9950541895712,-6.6067812144727,175.688231083653));
#13968=CARTESIAN_POINT('Ctrl Pts',(-54.9633937640365,-6.48434226598442,
176.556150922255));
#13969=CARTESIAN_POINT('Ctrl Pts',(-54.1573516980127,-6.0949735677162,177.812809342709));
#13970=CARTESIAN_POINT('Ctrl Pts',(-53.3979887985791,-5.83073710308303,
178.172806822259));
#13971=CARTESIAN_POINT('Ctrl Pts',(-51.9519097716579,-5.31810666795101,
177.994568269632));
#13972=CARTESIAN_POINT('Ctrl Pts',(-51.2952074816856,-5.0735953089356,177.458800517348));
#13973=CARTESIAN_POINT('Ctrl Pts',(-50.7993635736617,-4.74342220821161,
176.031468409862));
#13974=CARTESIAN_POINT('Ctrl Pts',(-50.9692613848378,-4.65940397939939,
175.170313217647));
#13975=CARTESIAN_POINT('Ctrl Pts',(-52.0040245669764,-4.62293999106357,
174.01934301833));
#13976=CARTESIAN_POINT('Ctrl Pts',(-52.8385688131003,-4.66759138415716,
173.754231358386));
#13977=CARTESIAN_POINT('Ctrl Pts',(-54.3414847379305,-4.72329909029368,
174.103969484305));
#13978=CARTESIAN_POINT('Ctrl Pts',(-54.9761466933045,-4.72791014175074,
174.714716972292));
#13979=CARTESIAN_POINT('Ctrl Pts',(-55.3975165431988,-4.57549651155636,
176.192173272167));
#13980=CARTESIAN_POINT('Ctrl Pts',(-55.1760506072609,-4.4148786220368,177.03103539143));
#13981=CARTESIAN_POINT('Ctrl Pts',(-54.1093043232961,-3.97451188101218,
178.061753391873));
#13982=CARTESIAN_POINT('Ctrl Pts',(-53.2902925544343,-3.69995792969149,
178.233822626392));
#13983=CARTESIAN_POINT('Ctrl Pts',(-51.9203920380846,-3.19963469730891,
177.711493690972));
#13984=CARTESIAN_POINT('Ctrl Pts',(-51.4044324721558,-2.98383265912278,
177.036002564632));
#13985=CARTESIAN_POINT('Ctrl Pts',(-51.237949425703,-2.71774512370317,175.525044339462));
#13986=CARTESIAN_POINT('Ctrl Pts',(-51.5957499271559,-2.66894330374766,
174.721509320474));
#13987=CARTESIAN_POINT('Ctrl Pts',(-52.8541051305037,-2.67783999801612,
173.825937213487));
#13988=CARTESIAN_POINT('Ctrl Pts',(-53.7315999697276,-2.7292086653859,173.7525048498));
#13989=CARTESIAN_POINT('Ctrl Pts',(-55.1208667949195,-2.76252327401043,
174.431246184642));
#13990=CARTESIAN_POINT('Ctrl Pts',(-55.6054709668258,-2.73893798071373,
175.167402226862));
#13991=CARTESIAN_POINT('Ctrl Pts',(-55.6603171863937,-2.58869274068622,
176.211840888345));
#13992=CARTESIAN_POINT('Ctrl Pts',(-55.6210463302226,-2.5392081864434,176.490448482462));
#13993=CARTESIAN_POINT('Ctrl Pts',(-55.4836397365907,-2.4479441182576,176.880586390838));
#13994=CARTESIAN_POINT('Ctrl Pts',(-55.4253285390117,-2.41535251334816,
177.005027857449));
#13995=CARTESIAN_POINT('Ctrl Pts',(-55.321414213033,-2.36345060131236,177.180440236558));
#13996=CARTESIAN_POINT('Ctrl Pts',(-55.2840225057543,-2.34563722905757,
177.23703696138));
#13997=CARTESIAN_POINT('Ctrl Pts',(-55.2039936793606,-2.30896761153951,
177.345998347345));
#13998=CARTESIAN_POINT('Ctrl Pts',(-55.1587206712145,-2.28906361698866,
177.401367187303));
#13999=CARTESIAN_POINT('Ctrl Pts',(-55.1161897096451,-2.27071607222657,
177.448351373365));
#14000=CARTESIAN_POINT('Ctrl Pts',(-47.8886718415116,-31.6995536639001,
175.585485069079));
#14001=CARTESIAN_POINT('Ctrl Pts',(-47.9424090991571,-31.4208895534118,
175.585485069079));
#14002=CARTESIAN_POINT('Ctrl Pts',(-48.0165136638412,-31.142217631488,175.587595470504));
#14003=CARTESIAN_POINT('Ctrl Pts',(-48.206190379979,-30.6092681473582,175.5992945923));
#14004=CARTESIAN_POINT('Ctrl Pts',(-48.3219855416571,-30.3543443720961,
175.608895409754));
#14005=CARTESIAN_POINT('Ctrl Pts',(-48.7193595355016,-29.6463117438825,
175.654781597023));
#14006=CARTESIAN_POINT('Ctrl Pts',(-49.0545911241397,-29.252967076522,175.707428551708));
#14007=CARTESIAN_POINT('Ctrl Pts',(-49.5445318563166,-28.7861739714513,
175.852028081795));
#14008=CARTESIAN_POINT('Ctrl Pts',(-49.6987397911889,-28.6436248452838,
175.911397856293));
#14009=CARTESIAN_POINT('Ctrl Pts',(-49.9262155871255,-28.4691236019893,
176.025260422827));
#14010=CARTESIAN_POINT('Ctrl Pts',(-50.0186861454797,-28.4371266816906,
176.06691518842));
#14011=CARTESIAN_POINT('Ctrl Pts',(-50.1842299781189,-28.3689363752761,
176.173317219728));
#14012=CARTESIAN_POINT('Ctrl Pts',(-50.2569026354171,-28.3307458842207,
176.235836425973));
#14013=CARTESIAN_POINT('Ctrl Pts',(-50.4390882192945,-28.20291241382,176.455121758264));
#14014=CARTESIAN_POINT('Ctrl Pts',(-50.5079392950738,-28.0960057551614,
176.657103040121));
#14015=CARTESIAN_POINT('Ctrl Pts',(-50.4672993044493,-27.9634501974094,
176.968869644582));
#14016=CARTESIAN_POINT('Ctrl Pts',(-50.4326818607288,-27.9245995634275,
177.070967051899));
#14017=CARTESIAN_POINT('Ctrl Pts',(-50.3339110252539,-27.8569369682875,
177.264936028611));
#14018=CARTESIAN_POINT('Ctrl Pts',(-50.2683927599471,-27.8299386004748,
177.362186354007));
#14019=CARTESIAN_POINT('Ctrl Pts',(-50.193114320713,-27.8005016688432,177.448440461337));
#14020=CARTESIAN_POINT('Ctrl Pts',(-47.1031441589869,-31.5480734342088,
175.585485069079));
#14021=CARTESIAN_POINT('Ctrl Pts',(-47.1603662041614,-31.2513383379729,
175.585485069079));
#14022=CARTESIAN_POINT('Ctrl Pts',(-47.2482359974308,-30.9149655772776,
175.587875715227));
#14023=CARTESIAN_POINT('Ctrl Pts',(-47.4670950242505,-30.3000308864083,
175.601419934118));
#14024=CARTESIAN_POINT('Ctrl Pts',(-47.6018961077871,-30.0028542362142,
175.612574303893));
#14025=CARTESIAN_POINT('Ctrl Pts',(-48.06625584225,-29.1754899206181,175.666311941427));
#14026=CARTESIAN_POINT('Ctrl Pts',(-48.4618683742085,-28.7136853353929,
175.729732505271));
#14027=CARTESIAN_POINT('Ctrl Pts',(-49.0063756293611,-28.1949480459011,
175.890763292055));
#14028=CARTESIAN_POINT('Ctrl Pts',(-49.1677731230246,-28.0480163131157,
175.972468320302));
#14029=CARTESIAN_POINT('Ctrl Pts',(-49.3965343491423,-27.8703147335455,
176.056354650694));
#14030=CARTESIAN_POINT('Ctrl Pts',(-49.5042735598544,-27.8224509492496,
176.029622920355));
#14031=CARTESIAN_POINT('Ctrl Pts',(-49.714154138436,-27.7365778903946,176.021696276872));
#14032=CARTESIAN_POINT('Ctrl Pts',(-49.8092250008766,-27.6958009021663,
176.040400247712));
#14033=CARTESIAN_POINT('Ctrl Pts',(-50.0526599599857,-27.5670382667944,
176.149507116298));
#14034=CARTESIAN_POINT('Ctrl Pts',(-50.1573360552302,-27.4697774585579,
176.29868387691));
#14035=CARTESIAN_POINT('Ctrl Pts',(-50.1883082447542,-27.3362137867349,
176.557013250615));
#14036=CARTESIAN_POINT('Ctrl Pts',(-50.1794299894878,-27.2944646349798,
176.647304730812));
#14037=CARTESIAN_POINT('Ctrl Pts',(-50.1311335533471,-27.2163290407286,
176.829965813571));
#14038=CARTESIAN_POINT('Ctrl Pts',(-50.0905156624001,-27.1753600677279,
176.937389673553));
#14039=CARTESIAN_POINT('Ctrl Pts',(-50.0383214665825,-27.1440081492037,
177.018259765604));
#14040=CARTESIAN_POINT('Ctrl Pts',(-47.1031441589869,-31.5480734342088,
176.385485069079));
#14041=CARTESIAN_POINT('Ctrl Pts',(-47.1599854936771,-31.2533125799253,
176.385485069079));
#14042=CARTESIAN_POINT('Ctrl Pts',(-47.2462550636215,-30.9240508319461,
176.387855155919));
#14043=CARTESIAN_POINT('Ctrl Pts',(-47.460249087206,-30.3229192382893,176.401096636113));
#14044=CARTESIAN_POINT('Ctrl Pts',(-47.5913742255291,-30.0344018731676,
176.411980487031));
#14045=CARTESIAN_POINT('Ctrl Pts',(-48.0375122982338,-29.2397387684011,
176.463601555155));
#14046=CARTESIAN_POINT('Ctrl Pts',(-48.4124469809922,-28.8074108937189,
176.525602813253));
#14047=CARTESIAN_POINT('Ctrl Pts',(-48.8848496853331,-28.3577893519108,
176.665278154737));
#14048=CARTESIAN_POINT('Ctrl Pts',(-49.026848150992,-28.2513597906944,176.736022770841));
#14049=CARTESIAN_POINT('Ctrl Pts',(-49.1705854582322,-28.1079648662814,
176.786782875481));
#14050=CARTESIAN_POINT('Ctrl Pts',(-49.2060240792629,-28.0278386987345,
176.747088553392));
#14051=CARTESIAN_POINT('Ctrl Pts',(-49.2810889004422,-27.9003322593211,
176.67860791329));
#14052=CARTESIAN_POINT('Ctrl Pts',(-49.3144205003265,-27.8541778608178,
176.654181717029));
#14053=CARTESIAN_POINT('Ctrl Pts',(-49.3895778283813,-27.7529515714288,
176.588058724708));
#14054=CARTESIAN_POINT('Ctrl Pts',(-49.4143850760995,-27.7397337398683,
176.533088088996));
#14055=CARTESIAN_POINT('Ctrl Pts',(-49.4653959512805,-27.6892053509014,
176.504625861351));
#14056=CARTESIAN_POINT('Ctrl Pts',(-49.480846052191,-27.6666966453102,176.508814220202));
#14057=CARTESIAN_POINT('Ctrl Pts',(-49.4871117159947,-27.6078471194517,
176.551208753368));
#14058=CARTESIAN_POINT('Ctrl Pts',(-49.4794905861727,-27.5632681966532,
176.593760604048));
#14059=CARTESIAN_POINT('Ctrl Pts',(-49.4509304485228,-27.5317240793367,
176.63793339336));
#14060=CARTESIAN_POINT('Ctrl Pts',(-47.8886718415116,-31.6995536639001,
176.385485069079));
#14061=CARTESIAN_POINT('Ctrl Pts',(-47.9420283886728,-31.4228637953642,
176.385485069079));
#14062=CARTESIAN_POINT('Ctrl Pts',(-48.014532730032,-31.1513028861565,176.387574911196));
#14063=CARTESIAN_POINT('Ctrl Pts',(-48.1993444429345,-30.6321564992392,
176.398971294295));
#14064=CARTESIAN_POINT('Ctrl Pts',(-48.3114636593991,-30.3858920090494,
176.408301592892));
#14065=CARTESIAN_POINT('Ctrl Pts',(-48.6906159914853,-29.7105605916654,
176.452071210751));
#14066=CARTESIAN_POINT('Ctrl Pts',(-49.0051697309234,-29.3466926348484,
176.50329885969));
#14067=CARTESIAN_POINT('Ctrl Pts',(-49.4230059122887,-28.9490152774608,
176.626542944478));
#14068=CARTESIAN_POINT('Ctrl Pts',(-49.5578148191563,-28.8469683228627,
176.674952306832));
#14069=CARTESIAN_POINT('Ctrl Pts',(-49.7002666962155,-28.7067737347251,
176.755688647613));
#14070=CARTESIAN_POINT('Ctrl Pts',(-49.7204366648883,-28.6425144311754,
176.784380821457));
#14071=CARTESIAN_POINT('Ctrl Pts',(-49.7511647401251,-28.5326907442027,
176.830228856146));
#14072=CARTESIAN_POINT('Ctrl Pts',(-49.7620981348669,-28.4891228428723,
176.849617895289));
#14073=CARTESIAN_POINT('Ctrl Pts',(-49.7760060876902,-28.3888257184543,
176.893673366674));
#14074=CARTESIAN_POINT('Ctrl Pts',(-49.764988315943,-28.3659620364717,176.891507252207));
#14075=CARTESIAN_POINT('Ctrl Pts',(-49.7443870109756,-28.3164417615759,
176.916482255318));
#14076=CARTESIAN_POINT('Ctrl Pts',(-49.7340979234319,-28.2968315737579,
176.932476541289));
#14077=CARTESIAN_POINT('Ctrl Pts',(-49.6898891879014,-28.2484550470107,
176.986178968408));
#14078=CARTESIAN_POINT('Ctrl Pts',(-49.6573676837196,-28.2178467294001,
177.018557284502));
#14079=CARTESIAN_POINT('Ctrl Pts',(-49.6057233026532,-28.1882175989763,
177.068114089093));
#14080=CARTESIAN_POINT('Ctrl Pts',(-48.6741995240363,-31.8510338935913,
176.385485069079));
#14081=CARTESIAN_POINT('Ctrl Pts',(-48.7240712836685,-31.5924150108031,
176.385485069079));
#14082=CARTESIAN_POINT('Ctrl Pts',(-48.7828103964424,-31.3785549403669,
176.387294666473));
#14083=CARTESIAN_POINT('Ctrl Pts',(-48.9384397986629,-30.941393760189,176.396845952478));
#14084=CARTESIAN_POINT('Ctrl Pts',(-49.0315530932691,-30.7373821449313,
176.404622698753));
#14085=CARTESIAN_POINT('Ctrl Pts',(-49.3437196847369,-30.1813824149298,
176.440540866346));
#14086=CARTESIAN_POINT('Ctrl Pts',(-49.5978924808545,-29.8859743759779,
176.480994906127));
#14087=CARTESIAN_POINT('Ctrl Pts',(-49.9611621392443,-29.5402412030108,
176.587807734218));
#14088=CARTESIAN_POINT('Ctrl Pts',(-50.0887814873205,-29.442576855031,176.613881842823));
#14089=CARTESIAN_POINT('Ctrl Pts',(-50.2299479341988,-29.3055826031689,
176.724594419746));
#14090=CARTESIAN_POINT('Ctrl Pts',(-50.2348492505137,-29.2571901636164,
176.821673089522));
#14091=CARTESIAN_POINT('Ctrl Pts',(-50.221240579808,-29.1650492290843,176.981849799003));
#14092=CARTESIAN_POINT('Ctrl Pts',(-50.2097757694073,-29.1240678249268,
177.04505407355));
#14093=CARTESIAN_POINT('Ctrl Pts',(-50.162434346999,-29.0246998654798,177.199288008639));
#14094=CARTESIAN_POINT('Ctrl Pts',(-50.1155915557866,-28.9921903330752,
177.249926415417));
#14095=CARTESIAN_POINT('Ctrl Pts',(-50.0233780706706,-28.9436781722504,
177.328338649285));
#14096=CARTESIAN_POINT('Ctrl Pts',(-49.9873497946729,-28.9269665022055,
177.356138862376));
#14097=CARTESIAN_POINT('Ctrl Pts',(-49.8926666598081,-28.8890629745697,
177.421149183448));
#14098=CARTESIAN_POINT('Ctrl Pts',(-49.8352447812666,-28.872425262147,177.443353964955));
#14099=CARTESIAN_POINT('Ctrl Pts',(-49.7605161567837,-28.8447111186158,
177.498294784826));
#14100=CARTESIAN_POINT('Ctrl Pts',(-48.6741995240363,-31.8510338935913,
175.585485069079));
#14101=CARTESIAN_POINT('Ctrl Pts',(-48.7244519941528,-31.5904407688506,
175.585485069079));
#14102=CARTESIAN_POINT('Ctrl Pts',(-48.7847913302516,-31.3694696856984,
175.587315225781));
#14103=CARTESIAN_POINT('Ctrl Pts',(-48.9452857357075,-30.918505408308,175.597169250483));
#14104=CARTESIAN_POINT('Ctrl Pts',(-49.042074975527,-30.7058345079779,175.605216515615));
#14105=CARTESIAN_POINT('Ctrl Pts',(-49.3724632287533,-30.1171335671469,
175.643251252618));
#14106=CARTESIAN_POINT('Ctrl Pts',(-49.6473138740709,-29.7922488176511,
175.685124598145));
#14107=CARTESIAN_POINT('Ctrl Pts',(-50.0826880832722,-29.3773998970014,
175.813292871536));
#14108=CARTESIAN_POINT('Ctrl Pts',(-50.2297064593532,-29.239233377452,175.850327392284));
#14109=CARTESIAN_POINT('Ctrl Pts',(-50.4558968251088,-29.0679324704331,
175.99416619496));
#14110=CARTESIAN_POINT('Ctrl Pts',(-50.5330987311051,-29.0518024141316,
176.104207456485));
#14111=CARTESIAN_POINT('Ctrl Pts',(-50.6543058178018,-29.0012948601576,
176.324938162585));
#14112=CARTESIAN_POINT('Ctrl Pts',(-50.7045802699575,-28.9656908662752,
176.431272604233));
#14113=CARTESIAN_POINT('Ctrl Pts',(-50.8255164786033,-28.8387865608456,
176.760736400229));
#14114=CARTESIAN_POINT('Ctrl Pts',(-50.8585425349173,-28.722234051765,177.015522203332));
#14115=CARTESIAN_POINT('Ctrl Pts',(-50.7462903641443,-28.5906866080838,
177.38072603855));
#14116=CARTESIAN_POINT('Ctrl Pts',(-50.6859337319697,-28.5547344918753,
177.494629372986));
#14117=CARTESIAN_POINT('Ctrl Pts',(-50.5366884971606,-28.4975448958465,
177.699906243651));
#14118=CARTESIAN_POINT('Ctrl Pts',(-50.446269857494,-28.4845171332217,177.786983034461));
#14119=CARTESIAN_POINT('Ctrl Pts',(-50.3479071748434,-28.4569951884828,
177.87862115707));
#14120=CARTESIAN_POINT('Ctrl Pts',(-47.8886718415116,-31.6995536639001,
175.585485069079));
#14121=CARTESIAN_POINT('Ctrl Pts',(-47.9424090991571,-31.4208895534118,
175.585485069079));
#14122=CARTESIAN_POINT('Ctrl Pts',(-48.0165136638412,-31.142217631488,175.587595470504));
#14123=CARTESIAN_POINT('Ctrl Pts',(-48.206190379979,-30.6092681473582,175.5992945923));
#14124=CARTESIAN_POINT('Ctrl Pts',(-48.3219855416571,-30.3543443720961,
175.608895409754));
#14125=CARTESIAN_POINT('Ctrl Pts',(-48.7193595355016,-29.6463117438825,
175.654781597023));
#14126=CARTESIAN_POINT('Ctrl Pts',(-49.0545911241397,-29.252967076522,175.707428551708));
#14127=CARTESIAN_POINT('Ctrl Pts',(-49.5445318563166,-28.7861739714513,
175.852028081795));
#14128=CARTESIAN_POINT('Ctrl Pts',(-49.6987397911889,-28.6436248452838,
175.911397856293));
#14129=CARTESIAN_POINT('Ctrl Pts',(-49.9262155871255,-28.4691236019893,
176.025260422827));
#14130=CARTESIAN_POINT('Ctrl Pts',(-50.0186861454797,-28.4371266816906,
176.06691518842));
#14131=CARTESIAN_POINT('Ctrl Pts',(-50.1842299781189,-28.3689363752761,
176.173317219728));
#14132=CARTESIAN_POINT('Ctrl Pts',(-50.2569026354171,-28.3307458842207,
176.235836425973));
#14133=CARTESIAN_POINT('Ctrl Pts',(-50.4390882192945,-28.20291241382,176.455121758264));
#14134=CARTESIAN_POINT('Ctrl Pts',(-50.5079392950738,-28.0960057551614,
176.657103040121));
#14135=CARTESIAN_POINT('Ctrl Pts',(-50.4672993044493,-27.9634501974094,
176.968869644582));
#14136=CARTESIAN_POINT('Ctrl Pts',(-50.4326818607288,-27.9245995634275,
177.070967051899));
#14137=CARTESIAN_POINT('Ctrl Pts',(-50.3339110252539,-27.8569369682875,
177.264936028611));
#14138=CARTESIAN_POINT('Ctrl Pts',(-50.2683927599471,-27.8299386004748,
177.362186354007));
#14139=CARTESIAN_POINT('Ctrl Pts',(-50.193114320713,-27.8005016688432,177.448440461337));
#14140=CARTESIAN_POINT('',(-47.8886718415116,-31.6995536639001,176.385485069079));
#14141=CARTESIAN_POINT('',(-47.8886718415116,-31.6995536639001,175.585485069079));
#14142=CARTESIAN_POINT('Origin',(-47.8886718415116,-31.6995536639001,175.985485069079));
#14143=CARTESIAN_POINT('Ctrl Pts',(-47.8886718415116,-31.6995536639001,
176.385485069079));
#14144=CARTESIAN_POINT('Ctrl Pts',(-47.9420283886728,-31.4228637953642,
176.385485069079));
#14145=CARTESIAN_POINT('Ctrl Pts',(-48.014532730032,-31.1513028861565,176.387574911196));
#14146=CARTESIAN_POINT('Ctrl Pts',(-48.1993444429345,-30.6321564992392,
176.398971294295));
#14147=CARTESIAN_POINT('Ctrl Pts',(-48.3114636593991,-30.3858920090494,
176.408301592892));
#14148=CARTESIAN_POINT('Ctrl Pts',(-48.6906159914853,-29.7105605916654,
176.452071210751));
#14149=CARTESIAN_POINT('Ctrl Pts',(-49.0051697309234,-29.3466926348484,
176.50329885969));
#14150=CARTESIAN_POINT('Ctrl Pts',(-49.4230059122887,-28.9490152774608,
176.626542944478));
#14151=CARTESIAN_POINT('Ctrl Pts',(-49.5578148191563,-28.8469683228627,
176.674952306832));
#14152=CARTESIAN_POINT('Ctrl Pts',(-49.7002666962155,-28.7067737347251,
176.755688647613));
#14153=CARTESIAN_POINT('Ctrl Pts',(-49.7204366648883,-28.6425144311754,
176.784380821457));
#14154=CARTESIAN_POINT('Ctrl Pts',(-49.7511647401251,-28.5326907442027,
176.830228856146));
#14155=CARTESIAN_POINT('Ctrl Pts',(-49.7620981348669,-28.4891228428723,
176.849617895289));
#14156=CARTESIAN_POINT('Ctrl Pts',(-49.7760060876902,-28.3888257184543,
176.893673366674));
#14157=CARTESIAN_POINT('Ctrl Pts',(-49.764988315943,-28.3659620364717,176.891507252207));
#14158=CARTESIAN_POINT('Ctrl Pts',(-49.7443870109756,-28.3164417615759,
176.916482255318));
#14159=CARTESIAN_POINT('Ctrl Pts',(-49.7340979234319,-28.2968315737579,
176.932476541289));
#14160=CARTESIAN_POINT('Ctrl Pts',(-49.6898891879014,-28.2484550470107,
176.986178968408));
#14161=CARTESIAN_POINT('Ctrl Pts',(-49.6573676837196,-28.2178467294001,
177.018557284502));
#14162=CARTESIAN_POINT('Ctrl Pts',(-49.6057233026533,-28.1882175989763,
177.068114089093));
#14163=CARTESIAN_POINT('Ctrl Pts',(-47.8886718415116,-31.6995536639001,
175.585485069079));
#14164=CARTESIAN_POINT('Ctrl Pts',(-47.9424090991571,-31.4208895534118,
175.585485069079));
#14165=CARTESIAN_POINT('Ctrl Pts',(-48.0165136638412,-31.142217631488,175.587595470504));
#14166=CARTESIAN_POINT('Ctrl Pts',(-48.206190379979,-30.6092681473582,175.5992945923));
#14167=CARTESIAN_POINT('Ctrl Pts',(-48.3219855416571,-30.3543443720961,
175.608895409754));
#14168=CARTESIAN_POINT('Ctrl Pts',(-48.7193595355016,-29.6463117438825,
175.654781597023));
#14169=CARTESIAN_POINT('Ctrl Pts',(-49.0545911241397,-29.252967076522,175.707428551708));
#14170=CARTESIAN_POINT('Ctrl Pts',(-49.5445318563166,-28.7861739714513,
175.852028081795));
#14171=CARTESIAN_POINT('Ctrl Pts',(-49.6987397911889,-28.6436248452838,
175.911397856293));
#14172=CARTESIAN_POINT('Ctrl Pts',(-49.9262155871255,-28.4691236019893,
176.025260422827));
#14173=CARTESIAN_POINT('Ctrl Pts',(-50.0186861454797,-28.4371266816906,
176.06691518842));
#14174=CARTESIAN_POINT('Ctrl Pts',(-50.1842299781189,-28.3689363752761,
176.173317219728));
#14175=CARTESIAN_POINT('Ctrl Pts',(-50.2569026354171,-28.3307458842207,
176.235836425973));
#14176=CARTESIAN_POINT('Ctrl Pts',(-50.4390882192945,-28.20291241382,176.455121758264));
#14177=CARTESIAN_POINT('Ctrl Pts',(-50.5079392950738,-28.0960057551614,
176.657103040121));
#14178=CARTESIAN_POINT('Ctrl Pts',(-50.4672993044493,-27.9634501974094,
176.968869644582));
#14179=CARTESIAN_POINT('Ctrl Pts',(-50.4326818607288,-27.9245995634275,
177.070967051899));
#14180=CARTESIAN_POINT('Ctrl Pts',(-50.3339110252539,-27.8569369682875,
177.264936028611));
#14181=CARTESIAN_POINT('Ctrl Pts',(-50.2683927599471,-27.8299386004748,
177.362186354007));
#14182=CARTESIAN_POINT('Ctrl Pts',(-50.193114320713,-27.8005016688432,177.448440461337));
#14183=CARTESIAN_POINT('Origin',(-47.8413342697331,-31.9450310646891,175.985485069079));
#14184=CARTESIAN_POINT('',(-47.8413342697331,-31.9450310646891,175.585485069079));
#14185=CARTESIAN_POINT('Origin',(-47.8886718415116,-31.6995536639001,175.985485069079));
#14186=CARTESIAN_POINT('Ctrl Pts',(-55.1161897096451,-2.27071607222657,
177.448351373365));
#14187=CARTESIAN_POINT('Ctrl Pts',(-55.0544324803005,-2.24407445661358,
177.516574922684));
#14188=CARTESIAN_POINT('Ctrl Pts',(-55.0031840696463,-2.2159075942787,177.564829510218));
#14189=CARTESIAN_POINT('Ctrl Pts',(-54.8981614763103,-2.14735807337978,
177.649345866972));
#14190=CARTESIAN_POINT('Ctrl Pts',(-54.848196955649,-2.10845499517373,177.68122338125));
#14191=CARTESIAN_POINT('Ctrl Pts',(-54.7062455015458,-1.97869616397794,
177.747598981208));
#14192=CARTESIAN_POINT('Ctrl Pts',(-54.6230552819493,-1.87505607340526,
177.751980177594));
#14193=CARTESIAN_POINT('Ctrl Pts',(-54.4781164600507,-1.64599936204779,
177.704020550018));
#14194=CARTESIAN_POINT('Ctrl Pts',(-54.4161687409529,-1.52036398038793,
177.652507519121));
#14195=CARTESIAN_POINT('Ctrl Pts',(-54.3240884061122,-1.31623292778147,
177.552502738263));
#14196=CARTESIAN_POINT('Ctrl Pts',(-54.2900300114527,-1.2450809441322,177.5168693343));
#14197=CARTESIAN_POINT('Ctrl Pts',(-54.2388806708887,-1.10092476185966,
177.429650782512));
#14198=CARTESIAN_POINT('Ctrl Pts',(-54.2230625419579,-1.02814126447079,
177.378422455576));
#14199=CARTESIAN_POINT('Ctrl Pts',(-54.1687570862725,-0.661100958902222,
177.107656526019));
#14200=CARTESIAN_POINT('Ctrl Pts',(-54.1632550913909,-0.344986943697024,
176.855601626641));
#14201=CARTESIAN_POINT('Ctrl Pts',(-54.1894883174704,0.100428951784895,
176.57062132681));
#14202=CARTESIAN_POINT('Ctrl Pts',(-54.2038650968969,0.243821813285216,
176.491645489995));
#14203=CARTESIAN_POINT('Ctrl Pts',(-54.2289503028814,0.435912884592043,
176.413053638658));
#14204=CARTESIAN_POINT('Ctrl Pts',(-54.2378694870404,0.495988408430007,
176.393461416067));
#14205=CARTESIAN_POINT('Ctrl Pts',(-54.2511575637744,0.57777536525398,176.374426535183));
#14206=CARTESIAN_POINT('Ctrl Pts',(-54.2555861991508,0.603644576350343,
176.369782059628));
#14207=CARTESIAN_POINT('Ctrl Pts',(-54.2642818917577,0.652365455860021,
176.363705099944));
#14208=CARTESIAN_POINT('Ctrl Pts',(-54.2669281652524,0.666814619551347,
176.362269083675));
#14209=CARTESIAN_POINT('Ctrl Pts',(-54.2726708967805,0.696594575640996,
176.362269083675));
#14210=CARTESIAN_POINT('Ctrl Pts',(-54.9611536226478,-1.61438316700751,
177.018013216499));
#14211=CARTESIAN_POINT('Ctrl Pts',(-54.9292844549615,-1.59689979741686,
177.061501366048));
#14212=CARTESIAN_POINT('Ctrl Pts',(-54.9347169869457,-1.59513306644644,
177.059466012753));
#14213=CARTESIAN_POINT('Ctrl Pts',(-54.9393829236175,-1.59207559169288,
177.070205982371));
#14214=CARTESIAN_POINT('Ctrl Pts',(-54.9521671405265,-1.59794122115585,
177.067981920184));
#14215=CARTESIAN_POINT('Ctrl Pts',(-55.0007420885566,-1.63157855374127,
177.067321317852));
#14216=CARTESIAN_POINT('Ctrl Pts',(-55.035179086296,-1.66960295600012,177.085015349648));
#14217=CARTESIAN_POINT('Ctrl Pts',(-55.0396054390644,-1.63669166623166,
177.119603765033));
#14218=CARTESIAN_POINT('Ctrl Pts',(-55.0210115508064,-1.57122240422777,
177.125346825549));
#14219=CARTESIAN_POINT('Ctrl Pts',(-54.9916258301057,-1.40601129473046,
177.119012727072));
#14220=CARTESIAN_POINT('Ctrl Pts',(-54.9808143890584,-1.33515491542406,
177.122292216748));
#14221=CARTESIAN_POINT('Ctrl Pts',(-54.95716312305,-1.20146912437994,177.090609934045));
#14222=CARTESIAN_POINT('Ctrl Pts',(-54.9459301778233,-1.14025139494389,
177.054154311007));
#14223=CARTESIAN_POINT('Ctrl Pts',(-54.9010485418089,-0.837221085805294,
176.830475957374));
#14224=CARTESIAN_POINT('Ctrl Pts',(-54.8933924651384,-0.543523047070829,
176.59567568837));
#14225=CARTESIAN_POINT('Ctrl Pts',(-54.9188659939004,-0.109419407590943,
176.317655840143));
#14226=CARTESIAN_POINT('Ctrl Pts',(-54.9330773739472,0.0346181647599921,
176.23753447689));
#14227=CARTESIAN_POINT('Ctrl Pts',(-54.9598081399055,0.239682185419695,
176.153510553493));
#14228=CARTESIAN_POINT('Ctrl Pts',(-54.9696067027056,0.306181698359097,
176.131488679163));
#14229=CARTESIAN_POINT('Ctrl Pts',(-54.985167831776,0.402075433542801,176.109129772912));
#14230=CARTESIAN_POINT('Ctrl Pts',(-54.9905018003277,0.433390482627809,
176.103410426781));
#14231=CARTESIAN_POINT('Ctrl Pts',(-55.0013966992521,0.494658609580997,
176.095691012754));
#14232=CARTESIAN_POINT('Ctrl Pts',(-55.0061011366799,0.520171112552638,
176.093689066957));
#14233=CARTESIAN_POINT('Ctrl Pts',(-55.012606581275,0.553906252953576,176.093689066957));
#14234=CARTESIAN_POINT('Ctrl Pts',(-54.3738267566562,-2.00237092626598,
176.637865020199));
#14235=CARTESIAN_POINT('Ctrl Pts',(-54.3525463517218,-1.98561856641678,
176.665739674622));
#14236=CARTESIAN_POINT('Ctrl Pts',(-54.3544769039845,-1.9794317280201,176.664843524849));
#14237=CARTESIAN_POINT('Ctrl Pts',(-54.3701639946021,-1.97656111293176,
176.660021126843));
#14238=CARTESIAN_POINT('Ctrl Pts',(-54.3898340629218,-1.98406009722412,
176.649873028566));
#14239=CARTESIAN_POINT('Ctrl Pts',(-54.4615150878692,-2.02680400188237,
176.627416363355));
#14240=CARTESIAN_POINT('Ctrl Pts',(-54.5129888400511,-2.0757703324506,176.634526145744));
#14241=CARTESIAN_POINT('Ctrl Pts',(-54.5552784049148,-2.06122690211322,
176.64442773024));
#14242=CARTESIAN_POINT('Ctrl Pts',(-54.5578076149692,-2.0038135240127,176.634785085717));
#14243=CARTESIAN_POINT('Ctrl Pts',(-54.5892177302657,-1.85411233048761,
176.591889300217));
#14244=CARTESIAN_POINT('Ctrl Pts',(-54.610530702465,-1.78996529622254,176.577740776828));
#14245=CARTESIAN_POINT('Ctrl Pts',(-54.6268123436843,-1.66507238716025,
176.528080652247));
#14246=CARTESIAN_POINT('Ctrl Pts',(-54.6208424301061,-1.60549754243094,
176.490359176158));
#14247=CARTESIAN_POINT('Ctrl Pts',(-54.5752745689856,-1.29850461246565,
176.263815183543));
#14248=CARTESIAN_POINT('Ctrl Pts',(-54.5643152196599,-0.983878310891091,
176.010083812441));
#14249=CARTESIAN_POINT('Ctrl Pts',(-54.5948528025329,-0.459382509277473,
175.674365954678));
#14250=CARTESIAN_POINT('Ctrl Pts',(-54.6123879900288,-0.274694122222572,
175.56925971577));
#14251=CARTESIAN_POINT('Ctrl Pts',(-54.6518354905867,0.0289042342998165,
175.444989413561));
#14252=CARTESIAN_POINT('Ctrl Pts',(-54.6672255747517,0.134792609497288,
175.409177545969));
#14253=CARTESIAN_POINT('Ctrl Pts',(-54.6945480274656,0.303452837912914,
175.369907772329));
#14254=CARTESIAN_POINT('Ctrl Pts',(-54.7043366789371,0.361315642399545,
175.359237745269));
#14255=CARTESIAN_POINT('Ctrl Pts',(-54.7254408307236,0.480524258303587,
175.344341053851));
#14256=CARTESIAN_POINT('Ctrl Pts',(-54.7391421008419,0.554236948300629,
175.340121037765));
#14257=CARTESIAN_POINT('Ctrl Pts',(-54.7488852836436,0.604761956232279,
175.340121037765));
#14258=CARTESIAN_POINT('Ctrl Pts',(-54.5288628436534,-2.65870383148503,
177.068203177065));
#14259=CARTESIAN_POINT('Ctrl Pts',(-54.4776943770608,-2.6327932256135,177.120813231257));
#14260=CARTESIAN_POINT('Ctrl Pts',(-54.4229439866851,-2.60020625585236,
177.170207022314));
#14261=CARTESIAN_POINT('Ctrl Pts',(-54.3289425472948,-2.53184359461866,
177.239161011444));
#14262=CARTESIAN_POINT('Ctrl Pts',(-54.2858638780443,-2.494573871242,177.263114489632));
#14263=CARTESIAN_POINT('Ctrl Pts',(-54.1670185008584,-2.37392161211904,
177.307694026711));
#14264=CARTESIAN_POINT('Ctrl Pts',(-54.1008650357044,-2.28122344985573,
177.30149097369));
#14265=CARTESIAN_POINT('Ctrl Pts',(-53.9937894259011,-2.07053459792936,
177.228844515225));
#14266=CARTESIAN_POINT('Ctrl Pts',(-53.9529648051158,-1.95295510017287,
177.161945779289));
#14267=CARTESIAN_POINT('Ctrl Pts',(-53.9216803062721,-1.76433396353862,
177.025379311408));
#14268=CARTESIAN_POINT('Ctrl Pts',(-53.9197463248593,-1.6998913249307,176.97231789438));
#14269=CARTESIAN_POINT('Ctrl Pts',(-53.9085298915231,-1.56452802463996,
176.867121500714));
#14270=CARTESIAN_POINT('Ctrl Pts',(-53.8979747942407,-1.4933874119578,176.814627320727));
#14271=CARTESIAN_POINT('Ctrl Pts',(-53.8429831134493,-1.12238448556273,
176.540995752188));
#14272=CARTESIAN_POINT('Ctrl Pts',(-53.8341778459125,-0.785342207517119,
176.270009750712));
#14273=CARTESIAN_POINT('Ctrl Pts',(-53.8654751261029,-0.249534149901716,
175.927331441344));
#14274=CARTESIAN_POINT('Ctrl Pts',(-53.8831757129786,-0.0654904736973553,
175.823370728875));
#14275=CARTESIAN_POINT('Ctrl Pts',(-53.9209776535626,0.225134933472168,
175.704532498726));
#14276=CARTESIAN_POINT('Ctrl Pts',(-53.9354883590865,0.324599319568198,
175.671150282872));
#14277=CARTESIAN_POINT('Ctrl Pts',(-53.960537759464,0.479152769624093,175.6352045346));
#14278=CARTESIAN_POINT('Ctrl Pts',(-53.9694210777602,0.531569736122078,
175.625609378116));
#14279=CARTESIAN_POINT('Ctrl Pts',(-53.9883260232292,0.638231104582612,
175.612355141042));
#14280=CARTESIAN_POINT('Ctrl Pts',(-53.9999691294144,0.700880455299337,
175.608701054484));
#14281=CARTESIAN_POINT('Ctrl Pts',(-54.0089495991491,0.747450278919698,
175.608701054484));
#14282=CARTESIAN_POINT('Ctrl Pts',(-54.6838989306507,-3.31503673670408,
177.498541333932));
#14283=CARTESIAN_POINT('Ctrl Pts',(-54.6028424023999,-3.27996788481022,
177.575886787893));
#14284=CARTESIAN_POINT('Ctrl Pts',(-54.4914110693857,-3.22098078368462,
177.675570519779));
#14285=CARTESIAN_POINT('Ctrl Pts',(-54.2877210999876,-3.08712607630556,
177.818300896045));
#14286=CARTESIAN_POINT('Ctrl Pts',(-54.1818936931668,-3.00508764525988,
177.876355950698));
#14287=CARTESIAN_POINT('Ctrl Pts',(-53.8725219138475,-2.7210392223557,177.987971690067));
#14288=CARTESIAN_POINT('Ctrl Pts',(-53.6887412313577,-2.48667656726087,
177.968455801636));
#14289=CARTESIAN_POINT('Ctrl Pts',(-53.4323004468874,-2.07984229374549,
177.81326130021));
#14290=CARTESIAN_POINT('Ctrl Pts',(-53.3481219952623,-1.90209667633303,
177.689106472861));
#14291=CARTESIAN_POINT('Ctrl Pts',(-53.2541428822785,-1.67455559658963,
177.4588693226));
#14292=CARTESIAN_POINT('Ctrl Pts',(-53.2289619472537,-1.60981735363885,
177.366895011932));
#14293=CARTESIAN_POINT('Ctrl Pts',(-53.1902474393619,-1.46398366211967,
177.206162349181));
#14294=CARTESIAN_POINT('Ctrl Pts',(-53.1751071583752,-1.38127728148465,
177.138895465296));
#14295=CARTESIAN_POINT('Ctrl Pts',(-53.1106916579129,-0.946264358659819,
176.818176320833));
#14296=CARTESIAN_POINT('Ctrl Pts',(-53.104040472165,-0.586806104143147,
176.529935688984));
#14297=CARTESIAN_POINT('Ctrl Pts',(-53.1360974496729,-0.0396857905259603,
176.18029692801));
#14298=CARTESIAN_POINT('Ctrl Pts',(-53.1539634359283,0.143713174827862,
176.077481741979));
#14299=CARTESIAN_POINT('Ctrl Pts',(-53.1901198165385,0.421365632644519,
175.964075583891));
#14300=CARTESIAN_POINT('Ctrl Pts',(-53.2037511434212,0.514406029639107,
175.933123019776));
#14301=CARTESIAN_POINT('Ctrl Pts',(-53.2265274914624,0.654852701335273,
175.900501296871));
#14302=CARTESIAN_POINT('Ctrl Pts',(-53.2345054765832,0.701823829844612,
175.891981010963));
#14303=CARTESIAN_POINT('Ctrl Pts',(-53.2512112157347,0.795937950861637,
175.880369228233));
#14304=CARTESIAN_POINT('Ctrl Pts',(-53.2607961579869,0.847523962298047,
175.877281071202));
#14305=CARTESIAN_POINT('Ctrl Pts',(-53.2690139146546,0.890138601607118,
175.877281071202));
#14306=CARTESIAN_POINT('Ctrl Pts',(-55.2712257966423,-2.92704897744562,
177.878689530232));
#14307=CARTESIAN_POINT('Ctrl Pts',(-55.1795805056396,-2.8912491158103,177.971648479319));
#14308=CARTESIAN_POINT('Ctrl Pts',(-55.071651152347,-2.83668212211097,178.070193007683));
#14309=CARTESIAN_POINT('Ctrl Pts',(-54.8569400290031,-2.70264055506668,
178.228485751573));
#14310=CARTESIAN_POINT('Ctrl Pts',(-54.7442267707714,-2.61896876919161,
178.294464842316));
#14311=CARTESIAN_POINT('Ctrl Pts',(-54.411748914535,-2.3258137742146,178.427876644564));
#14312=CARTESIAN_POINT('Ctrl Pts',(-54.2109314776027,-2.08050919081039,
178.41894500554));
#14313=CARTESIAN_POINT('Ctrl Pts',(-53.916627481037,-1.65530705786393,178.288437335003));
#14314=CARTESIAN_POINT('Ctrl Pts',(-53.8113259310995,-1.4695055565481,178.179668212693));
#14315=CARTESIAN_POINT('Ctrl Pts',(-53.6565509821185,-1.22645456083248,
177.985992749455));
#14316=CARTESIAN_POINT('Ctrl Pts',(-53.5992456338471,-1.15500697284035,
177.911446451852));
#14317=CARTESIAN_POINT('Ctrl Pts',(-53.5205982187275,-1.00038039933938,
177.768691630978));
#14318=CARTESIAN_POINT('Ctrl Pts',(-53.5001949060925,-0.916031133997679,
177.702690600146));
#14319=CARTESIAN_POINT('Ctrl Pts',(-53.4364656307362,-0.484980831999149,
177.384837094664));
#14320=CARTESIAN_POINT('Ctrl Pts',(-53.4331177176434,-0.146450840323217,
177.115527564913));
#14321=CARTESIAN_POINT('Ctrl Pts',(-53.4601106410404,0.310277311160734,
176.823586813476));
#14322=CARTESIAN_POINT('Ctrl Pts',(-53.4746528198466,0.453025461810439,
176.745756503099));
#14323=CARTESIAN_POINT('Ctrl Pts',(-53.4980924658573,0.632143583764391,
176.672596723823));
#14324=CARTESIAN_POINT('Ctrl Pts',(-53.5061322713752,0.685795118500917,
176.65543415297));
#14325=CARTESIAN_POINT('Ctrl Pts',(-53.5171472957729,0.75347529696516,176.639723297454));
#14326=CARTESIAN_POINT('Ctrl Pts',(-53.5206705979738,0.773898670072877,
176.636153692475));
#14327=CARTESIAN_POINT('Ctrl Pts',(-53.5271670842632,0.810072302139046,
176.631719187135));
#14328=CARTESIAN_POINT('Ctrl Pts',(-53.5277551938249,0.813458126550056,
176.630849100393));
#14329=CARTESIAN_POINT('Ctrl Pts',(-53.532735212286,0.839282898328416,176.630849100393));
#14330=CARTESIAN_POINT('Ctrl Pts',(-55.1161897096451,-2.27071607222657,
177.448351373365));
#14331=CARTESIAN_POINT('Ctrl Pts',(-55.0544324803005,-2.24407445661358,
177.516574922684));
#14332=CARTESIAN_POINT('Ctrl Pts',(-55.0031840696463,-2.2159075942787,177.564829510218));
#14333=CARTESIAN_POINT('Ctrl Pts',(-54.8981614763103,-2.14735807337978,
177.649345866972));
#14334=CARTESIAN_POINT('Ctrl Pts',(-54.848196955649,-2.10845499517373,177.68122338125));
#14335=CARTESIAN_POINT('Ctrl Pts',(-54.7062455015458,-1.97869616397794,
177.747598981208));
#14336=CARTESIAN_POINT('Ctrl Pts',(-54.6230552819493,-1.87505607340526,
177.751980177594));
#14337=CARTESIAN_POINT('Ctrl Pts',(-54.4781164600507,-1.64599936204779,
177.704020550018));
#14338=CARTESIAN_POINT('Ctrl Pts',(-54.4161687409529,-1.52036398038793,
177.652507519121));
#14339=CARTESIAN_POINT('Ctrl Pts',(-54.3240884061122,-1.31623292778147,
177.552502738263));
#14340=CARTESIAN_POINT('Ctrl Pts',(-54.2900300114527,-1.2450809441322,177.5168693343));
#14341=CARTESIAN_POINT('Ctrl Pts',(-54.2388806708887,-1.10092476185966,
177.429650782512));
#14342=CARTESIAN_POINT('Ctrl Pts',(-54.2230625419579,-1.02814126447079,
177.378422455576));
#14343=CARTESIAN_POINT('Ctrl Pts',(-54.1687570862725,-0.661100958902222,
177.107656526019));
#14344=CARTESIAN_POINT('Ctrl Pts',(-54.1632550913909,-0.344986943697024,
176.855601626641));
#14345=CARTESIAN_POINT('Ctrl Pts',(-54.1894883174704,0.100428951784895,
176.57062132681));
#14346=CARTESIAN_POINT('Ctrl Pts',(-54.2038650968969,0.243821813285216,
176.491645489995));
#14347=CARTESIAN_POINT('Ctrl Pts',(-54.2289503028814,0.435912884592043,
176.413053638658));
#14348=CARTESIAN_POINT('Ctrl Pts',(-54.2378694870404,0.495988408430007,
176.393461416067));
#14349=CARTESIAN_POINT('Ctrl Pts',(-54.2511575637744,0.57777536525398,176.374426535183));
#14350=CARTESIAN_POINT('Ctrl Pts',(-54.2555861991508,0.603644576350343,
176.369782059628));
#14351=CARTESIAN_POINT('Ctrl Pts',(-54.2642818917577,0.652365455860021,
176.363705099944));
#14352=CARTESIAN_POINT('Ctrl Pts',(-54.2669281652524,0.666814619551347,
176.362269083675));
#14353=CARTESIAN_POINT('Ctrl Pts',(-54.2726708967805,0.696594575640996,
176.362269083675));
#14354=CARTESIAN_POINT('Origin',(-54.8225262766493,-2.4647099518558,177.258277275215));
#14355=CARTESIAN_POINT('Ctrl Pts',(-50.193114320713,-27.8005016688432,177.448440461337));
#14356=CARTESIAN_POINT('Ctrl Pts',(-50.1356777281885,-27.7780416249781,
177.514251363723));
#14357=CARTESIAN_POINT('Ctrl Pts',(-50.0768656935625,-27.751543311514,177.569181845458));
#14358=CARTESIAN_POINT('Ctrl Pts',(-49.9502510673185,-27.7006718917524,
177.678131488152));
#14359=CARTESIAN_POINT('Ctrl Pts',(-49.8836384545372,-27.6746069642733,
177.728584647058));
#14360=CARTESIAN_POINT('Ctrl Pts',(-49.6751767137455,-27.5945945456976,
177.866776279515));
#14361=CARTESIAN_POINT('Ctrl Pts',(-49.5241175159801,-27.5384622401806,
177.941191651987));
#14362=CARTESIAN_POINT('Ctrl Pts',(-49.052722448706,-27.3677108924734,178.102046365205));
#14363=CARTESIAN_POINT('Ctrl Pts',(-48.713006227557,-27.2491092781452,178.126053652285));
#14364=CARTESIAN_POINT('Ctrl Pts',(-47.7382795874562,-26.9019657740439,
177.942209528285));
#14365=CARTESIAN_POINT('Ctrl Pts',(-47.1597470877608,-26.6842880122364,
177.461567693823));
#14366=CARTESIAN_POINT('Ctrl Pts',(-46.658904710499,-26.3725604903201,176.179580952166));
#14367=CARTESIAN_POINT('Ctrl Pts',(-46.744016732095,-26.2835354545934,175.410971277798));
#14368=CARTESIAN_POINT('Ctrl Pts',(-47.5354179070377,-26.2224078706935,
174.242909311213));
#14369=CARTESIAN_POINT('Ctrl Pts',(-48.2245449656354,-26.2493771368743,
173.87343933243));
#14370=CARTESIAN_POINT('Ctrl Pts',(-49.6317089464608,-26.3060463238627,
173.871895146128));
#14371=CARTESIAN_POINT('Ctrl Pts',(-50.3230600395606,-26.332977077053,174.238655026377));
#14372=CARTESIAN_POINT('Ctrl Pts',(-51.1153496063116,-26.2743348509258,
175.387691644257));
#14373=CARTESIAN_POINT('Ctrl Pts',(-51.2096393582444,-26.1855070701005,
176.164686974611));
#14374=CARTESIAN_POINT('Ctrl Pts',(-50.7213268039385,-25.8775623946772,
177.442968877094));
#14375=CARTESIAN_POINT('Ctrl Pts',(-50.1473617008829,-25.6602454668112,
177.932812658479));
#14376=CARTESIAN_POINT('Ctrl Pts',(-48.8451246534299,-25.1962898596545,
178.190564242377));
#14377=CARTESIAN_POINT('Ctrl Pts',(-48.1356293396501,-24.9529458243571,
177.955714348281));
#14378=CARTESIAN_POINT('Ctrl Pts',(-47.2268076672755,-24.5631416907191,
176.954286183848));
#14379=CARTESIAN_POINT('Ctrl Pts',(-47.0395646158613,-24.4209960169422,
176.20954077848));
#14380=CARTESIAN_POINT('Ctrl Pts',(-47.370313215787,-24.2726666068476,174.855768290097));
#14381=CARTESIAN_POINT('Ctrl Pts',(-47.8845545017147,-24.265674947158,174.26583855031));
#14382=CARTESIAN_POINT('Ctrl Pts',(-49.1994460468846,-24.3046603227726,
173.764180115318));
#14383=CARTESIAN_POINT('Ctrl Pts',(-49.9762257647407,-24.3480555327739,
173.861039734223));
#14384=CARTESIAN_POINT('Ctrl Pts',(-51.1285193941288,-24.3574791486806,
174.66646218052));
#14385=CARTESIAN_POINT('Ctrl Pts',(-51.4882290443068,-24.3203491702665,
175.364132112564));
#14386=CARTESIAN_POINT('Ctrl Pts',(-51.4777341832408,-24.1036300286494,
176.755680066459));
#14387=CARTESIAN_POINT('Ctrl Pts',(-51.1141102527119,-23.9275319100486,
177.423612084264));
#14388=CARTESIAN_POINT('Ctrl Pts',(-49.9940329966114,-23.4994535030053,
178.148719290634));
#14389=CARTESIAN_POINT('Ctrl Pts',(-49.2531996565364,-23.2503850964097,
178.195074921104));
#14390=CARTESIAN_POINT('Ctrl Pts',(-48.0540724826088,-22.804580182732,177.607487959387));
#14391=CARTESIAN_POINT('Ctrl Pts',(-47.6174629086983,-22.6140260251447,
176.985139741962));
#14392=CARTESIAN_POINT('Ctrl Pts',(-47.4549919432363,-22.3698803060775,
175.609945370482));
#14393=CARTESIAN_POINT('Ctrl Pts',(-47.7329522193418,-22.3169255939418,
174.876470615888));
#14394=CARTESIAN_POINT('Ctrl Pts',(-48.8440385240951,-22.3059754149369,
173.902867041218));
#14395=CARTESIAN_POINT('Ctrl Pts',(-49.7035599970344,-22.3554674780819,
173.739637329099));
#14396=CARTESIAN_POINT('Ctrl Pts',(-51.1531706356154,-22.4011313967338,
174.265066374312));
#14397=CARTESIAN_POINT('Ctrl Pts',(-51.7115054154064,-22.3910761212842,
174.945624054023));
#14398=CARTESIAN_POINT('Ctrl Pts',(-51.9563259347572,-22.2045289991918,
176.459132103654));
#14399=CARTESIAN_POINT('Ctrl Pts',(-51.63765119649,-22.0251559400258,177.262331468575));
#14400=CARTESIAN_POINT('Ctrl Pts',(-50.4571461815608,-21.5627984935069,
178.149907937338));
#14401=CARTESIAN_POINT('Ctrl Pts',(-49.6222512854117,-21.2849471395443,
178.217719280236));
#14402=CARTESIAN_POINT('Ctrl Pts',(-48.3256452005116,-20.7988977065915,
177.525255091295));
#14403=CARTESIAN_POINT('Ctrl Pts',(-47.8935170509031,-20.5993012814682,
176.78942555283));
#14404=CARTESIAN_POINT('Ctrl Pts',(-47.9069259765589,-20.3679964193449,
175.264267840625));
#14405=CARTESIAN_POINT('Ctrl Pts',(-48.3565963500671,-20.33698501403,174.508050023486));
#14406=CARTESIAN_POINT('Ctrl Pts',(-49.7115395236169,-20.3645147337819,
173.767258025586));
#14407=CARTESIAN_POINT('Ctrl Pts',(-50.5919963646361,-20.4163759449694,
173.798730113887));
#14408=CARTESIAN_POINT('Ctrl Pts',(-51.8921615926268,-20.4324111199544,
174.637786957993));
#14409=CARTESIAN_POINT('Ctrl Pts',(-52.2870845316673,-20.391715494119,175.425932171935));
#14410=CARTESIAN_POINT('Ctrl Pts',(-52.1845249551972,-20.1359343420921,
176.949348485014));
#14411=CARTESIAN_POINT('Ctrl Pts',(-51.6978717551623,-19.9258306519252,
177.647217385389));
#14412=CARTESIAN_POINT('Ctrl Pts',(-50.3567743114224,-19.4332812849397,
178.229888643815));
#14413=CARTESIAN_POINT('Ctrl Pts',(-49.531482093434,-19.1564117811874,178.098575810452));
#14414=CARTESIAN_POINT('Ctrl Pts',(-48.4209526978951,-18.7085233315365,
177.123331466978));
#14415=CARTESIAN_POINT('Ctrl Pts',(-48.1597795720535,-18.5402167412103,
176.29718764283));
#14416=CARTESIAN_POINT('Ctrl Pts',(-48.5145782694716,-18.3739619700934,
174.800216258582));
#14417=CARTESIAN_POINT('Ctrl Pts',(-49.1216168980297,-18.3741927637648,
174.159897255644));
#14418=CARTESIAN_POINT('Ctrl Pts',(-50.6124880467131,-18.4256628314289,
173.74530968569));
#14419=CARTESIAN_POINT('Ctrl Pts',(-51.4570089590119,-18.472296203581,173.973986288395));
#14420=CARTESIAN_POINT('Ctrl Pts',(-52.5367755134872,-18.4465314340497,
175.076321400051));
#14421=CARTESIAN_POINT('Ctrl Pts',(-52.7461464663159,-18.3691716102472,
175.928004990245));
#14422=CARTESIAN_POINT('Ctrl Pts',(-52.3166330239091,-18.0526500335514,
177.376965544067));
#14423=CARTESIAN_POINT('Ctrl Pts',(-51.6857211698905,-17.8130496454,177.945754508989));
#14424=CARTESIAN_POINT('Ctrl Pts',(-50.2465394893753,-17.3007990625156,
178.194297846636));
#14425=CARTESIAN_POINT('Ctrl Pts',(-49.4703000985441,-17.0343670318334,
177.871754882023));
#14426=CARTESIAN_POINT('Ctrl Pts',(-48.6088763818932,-16.6321365971318,
176.648991214725));
#14427=CARTESIAN_POINT('Ctrl Pts',(-48.5409020769561,-16.5028432711256,
175.78526591443));
#14428=CARTESIAN_POINT('Ctrl Pts',(-49.2164515058916,-16.3991203888251,
174.401518908745));
#14429=CARTESIAN_POINT('Ctrl Pts',(-49.9496118192587,-16.4227354715302,
173.914202886417));
#14430=CARTESIAN_POINT('Ctrl Pts',(-51.4902606534728,-16.4861638259448,
173.836744887307));
#14431=CARTESIAN_POINT('Ctrl Pts',(-52.2697075969923,-16.5185243960147,
174.249627738192));
#14432=CARTESIAN_POINT('Ctrl Pts',(-53.0792623986938,-16.4399376212412,
175.566241461313));
#14433=CARTESIAN_POINT('Ctrl Pts',(-53.0958608617722,-16.3264383488088,
176.440260240546));
#14434=CARTESIAN_POINT('Ctrl Pts',(-52.3498924896565,-15.9464100326616,
177.743856795072));
#14435=CARTESIAN_POINT('Ctrl Pts',(-51.6136771994172,-15.6882407493956,
178.142477224647));
#14436=CARTESIAN_POINT('Ctrl Pts',(-50.1619939854693,-15.1743526813971,
178.045393567771));
#14437=CARTESIAN_POINT('Ctrl Pts',(-49.479535393056,-14.9249532161513,177.547481856475));
#14438=CARTESIAN_POINT('Ctrl Pts',(-48.9083003859244,-14.5811172796918,
176.154888290848));
#14439=CARTESIAN_POINT('Ctrl Pts',(-49.032687325759,-14.4872017268269,175.286386043965));
#14440=CARTESIAN_POINT('Ctrl Pts',(-50.002899927607,-14.4395306566209,174.08106638639));
#14441=CARTESIAN_POINT('Ctrl Pts',(-50.8258619899905,-14.4815667576624,
173.768688449528));
#14442=CARTESIAN_POINT('Ctrl Pts',(-52.3490472247602,-14.5391579602322,
174.044477097964));
#14443=CARTESIAN_POINT('Ctrl Pts',(-53.0108480437211,-14.5505369630929,
174.618897762295));
#14444=CARTESIAN_POINT('Ctrl Pts',(-53.508606726061,-14.41258118913,176.072854784516));
#14445=CARTESIAN_POINT('Ctrl Pts',(-53.3308496256547,-14.2605010523332,
176.92211652172));
#14446=CARTESIAN_POINT('Ctrl Pts',(-52.3234046589676,-13.8325238003689,
178.011250192421));
#14447=CARTESIAN_POINT('Ctrl Pts',(-51.5138129382755,-13.5585438056648,
178.229366209696));
#14448=CARTESIAN_POINT('Ctrl Pts',(-50.1182607249297,-13.0546721198729,
177.788098654291));
#14449=CARTESIAN_POINT('Ctrl Pts',(-49.5630188185408,-12.8308644828691,
177.140857971114));
#14450=CARTESIAN_POINT('Ctrl Pts',(-49.3219040202974,-12.5483689245281,
175.637957478437));
#14451=CARTESIAN_POINT('Ctrl Pts',(-49.6365594730894,-12.4926951709364,
174.821179942866));
#14452=CARTESIAN_POINT('Ctrl Pts',(-50.8450351424658,-12.4918253386163,
173.862170041067));
#14453=CARTESIAN_POINT('Ctrl Pts',(-51.7160671936879,-12.5420406725331,
173.742988789581));
#14454=CARTESIAN_POINT('Ctrl Pts',(-53.1380531234061,-12.5824907099911,
174.344563971126));
#14455=CARTESIAN_POINT('Ctrl Pts',(-53.661497991413,-12.565516429584,175.054752397452));
#14456=CARTESIAN_POINT('Ctrl Pts',(-53.8242077932451,-12.3622912981454,
176.579637740953));
#14457=CARTESIAN_POINT('Ctrl Pts',(-53.4635573374974,-12.1759538811977,
177.362604506387));
#14458=CARTESIAN_POINT('Ctrl Pts',(-52.2358756182636,-11.7031645393402,
178.179207046235));
#14459=CARTESIAN_POINT('Ctrl Pts',(-51.404471480006,-11.4266005921062,178.198059647233));
#14460=CARTESIAN_POINT('Ctrl Pts',(-50.1465877134854,-10.9499764840513,
177.440684540534));
#14461=CARTESIAN_POINT('Ctrl Pts',(-49.7512566691313,-10.7559713173261,
176.677961727673));
#14462=CARTESIAN_POINT('Ctrl Pts',(-49.8442980389787,-10.5402489724976,
175.152069846099));
#14463=CARTESIAN_POINT('Ctrl Pts',(-50.3336227209985,-10.5166703329192,
174.417963751365));
#14464=CARTESIAN_POINT('Ctrl Pts',(-51.729412313951,-10.5511670115394,173.750914008412));
#14465=CARTESIAN_POINT('Ctrl Pts',(-52.6055357660183,-10.6034581645062,
173.829125569603));
#14466=CARTESIAN_POINT('Ctrl Pts',(-53.8591972775733,-10.6090268187652,
174.739479897504));
#14467=CARTESIAN_POINT('Ctrl Pts',(-54.2075655427863,-10.559958422732,175.542285446703));
#14468=CARTESIAN_POINT('Ctrl Pts',(-54.0309723767407,-10.2919570312328,
177.05153449857));
#14469=CARTESIAN_POINT('Ctrl Pts',(-53.5065211660476,-10.0729835636969,
177.724885949439));
#14470=CARTESIAN_POINT('Ctrl Pts',(-52.1359327706082,-9.57501150980407,
178.231990439602));
#14471=CARTESIAN_POINT('Ctrl Pts',(-51.3168725161042,-9.29919601638729,
178.055337178134));
#14472=CARTESIAN_POINT('Ctrl Pts',(-50.258716477129,-8.86039345968628,177.014257444883));
#14473=CARTESIAN_POINT('Ctrl Pts',(-50.0419858596938,-8.70190296068798,
176.174822144773));
#14474=CARTESIAN_POINT('Ctrl Pts',(-50.4788136762356,-8.55014763089762,
174.697436550109));
#14475=CARTESIAN_POINT('Ctrl Pts',(-51.1165600370436,-8.55674976323144,
174.095019459488));
#14476=CARTESIAN_POINT('Ctrl Pts',(-52.6206590619166,-8.6128620697194,173.755704628284));
#14477=CARTESIAN_POINT('Ctrl Pts',(-53.456626592603,-8.65630954771657,174.029197443714));
#14478=CARTESIAN_POINT('Ctrl Pts',(-54.4781193003427,-8.6195332279715,175.187078119489));
#14479=CARTESIAN_POINT('Ctrl Pts',(-54.643602443466,-8.53353572012608,176.04949882023));
#14480=CARTESIAN_POINT('Ctrl Pts',(-54.1354947853707,-8.20096498746117,
177.472181687833));
#14481=CARTESIAN_POINT('Ctrl Pts',(-53.4760203027823,-7.95706608118669,
178.003825172765));
#14482=CARTESIAN_POINT('Ctrl Pts',(-52.0249165538012,-7.441132564782,178.167825277993));
#14483=CARTESIAN_POINT('Ctrl Pts',(-51.2723007652614,-7.17976116760829,
177.802466009854));
#14484=CARTESIAN_POINT('Ctrl Pts',(-50.4742318046734,-6.79179686888332,
176.539214575509));
#14485=CARTESIAN_POINT('Ctrl Pts',(-50.4508393849021,-6.66952799804251,
175.667365550039));
#14486=CARTESIAN_POINT('Ctrl Pts',(-51.1982775200671,-6.57992894303025,
174.318931761547));
#14487=CARTESIAN_POINT('Ctrl Pts',(-51.9567203354133,-6.60831910752051,
173.869388776842));
#14488=CARTESIAN_POINT('Ctrl Pts',(-53.5030461170827,-6.67180659392302,
173.876188814802));
#14489=CARTESIAN_POINT('Ctrl Pts',(-54.2579318048227,-6.70074853854407,
174.329266762268));
#14490=CARTESIAN_POINT('Ctrl Pts',(-54.9950541895712,-6.6067812144727,175.688231083653));
#14491=CARTESIAN_POINT('Ctrl Pts',(-54.9633937640365,-6.48434226598442,
176.556150922255));
#14492=CARTESIAN_POINT('Ctrl Pts',(-54.1573516980127,-6.0949735677162,177.812809342709));
#14493=CARTESIAN_POINT('Ctrl Pts',(-53.3979887985791,-5.83073710308303,
178.172806822259));
#14494=CARTESIAN_POINT('Ctrl Pts',(-51.9519097716579,-5.31810666795101,
177.994568269632));
#14495=CARTESIAN_POINT('Ctrl Pts',(-51.2952074816856,-5.0735953089356,177.458800517348));
#14496=CARTESIAN_POINT('Ctrl Pts',(-50.7993635736617,-4.74342220821161,
176.031468409862));
#14497=CARTESIAN_POINT('Ctrl Pts',(-50.9692613848378,-4.65940397939939,
175.170313217647));
#14498=CARTESIAN_POINT('Ctrl Pts',(-52.0040245669764,-4.62293999106357,
174.01934301833));
#14499=CARTESIAN_POINT('Ctrl Pts',(-52.8385688131003,-4.66759138415716,
173.754231358386));
#14500=CARTESIAN_POINT('Ctrl Pts',(-54.3414847379305,-4.72329909029368,
174.103969484305));
#14501=CARTESIAN_POINT('Ctrl Pts',(-54.9761466933045,-4.72791014175074,
174.714716972292));
#14502=CARTESIAN_POINT('Ctrl Pts',(-55.3975165431988,-4.57549651155636,
176.192173272167));
#14503=CARTESIAN_POINT('Ctrl Pts',(-55.1760506072609,-4.4148786220368,177.03103539143));
#14504=CARTESIAN_POINT('Ctrl Pts',(-54.1093043232961,-3.97451188101218,
178.061753391873));
#14505=CARTESIAN_POINT('Ctrl Pts',(-53.2902925544343,-3.69995792969149,
178.233822626392));
#14506=CARTESIAN_POINT('Ctrl Pts',(-51.9203920380846,-3.19963469730891,
177.711493690972));
#14507=CARTESIAN_POINT('Ctrl Pts',(-51.4044324721558,-2.98383265912278,
177.036002564632));
#14508=CARTESIAN_POINT('Ctrl Pts',(-51.237949425703,-2.71774512370317,175.525044339462));
#14509=CARTESIAN_POINT('Ctrl Pts',(-51.5957499271559,-2.66894330374766,
174.721509320474));
#14510=CARTESIAN_POINT('Ctrl Pts',(-52.8541051305037,-2.67783999801612,
173.825937213487));
#14511=CARTESIAN_POINT('Ctrl Pts',(-53.7315999697276,-2.7292086653859,173.7525048498));
#14512=CARTESIAN_POINT('Ctrl Pts',(-55.1208667949195,-2.76252327401043,
174.431246184642));
#14513=CARTESIAN_POINT('Ctrl Pts',(-55.6054709668258,-2.73893798071373,
175.167402226862));
#14514=CARTESIAN_POINT('Ctrl Pts',(-55.6603171863937,-2.58869274068622,
176.211840888345));
#14515=CARTESIAN_POINT('Ctrl Pts',(-55.6210463302226,-2.5392081864434,176.490448482462));
#14516=CARTESIAN_POINT('Ctrl Pts',(-55.4836397365907,-2.4479441182576,176.880586390838));
#14517=CARTESIAN_POINT('Ctrl Pts',(-55.4253285390117,-2.41535251334816,
177.005027857449));
#14518=CARTESIAN_POINT('Ctrl Pts',(-55.321414213033,-2.36345060131236,177.180440236558));
#14519=CARTESIAN_POINT('Ctrl Pts',(-55.2840225057543,-2.34563722905757,
177.23703696138));
#14520=CARTESIAN_POINT('Ctrl Pts',(-55.2039936793606,-2.30896761153951,
177.345998347345));
#14521=CARTESIAN_POINT('Ctrl Pts',(-55.1587206712145,-2.28906361698866,
177.401367187303));
#14522=CARTESIAN_POINT('Ctrl Pts',(-55.1161897096451,-2.27071607222657,
177.448351373365));
#14523=CARTESIAN_POINT('Ctrl Pts',(-50.0383214665825,-27.1440081492037,
177.018259765604));
#14524=CARTESIAN_POINT('Ctrl Pts',(-49.9984978891038,-27.1200869921306,
177.079962725598));
#14525=CARTESIAN_POINT('Ctrl Pts',(-49.9575055461974,-27.1020674615118,
177.117111982701));
#14526=CARTESIAN_POINT('Ctrl Pts',(-49.8677888002033,-27.0582153119246,
177.208150208202));
#14527=CARTESIAN_POINT('Ctrl Pts',(-49.8200811333233,-27.0356913176731,
177.250904604008));
#14528=CARTESIAN_POINT('Ctrl Pts',(-49.6696339972988,-26.9667169890279,
177.369319858048));
#14529=CARTESIAN_POINT('Ctrl Pts',(-49.5596041625372,-26.9190141211719,
177.434440092329));
#14530=CARTESIAN_POINT('Ctrl Pts',(-49.2118492777513,-26.7720570333375,
177.585359994682));
#14531=CARTESIAN_POINT('Ctrl Pts',(-48.9561313182544,-26.6696252716912,
177.624018992736));
#14532=CARTESIAN_POINT('Ctrl Pts',(-48.2061347626312,-26.3651189875991,
177.541325063495));
#14533=CARTESIAN_POINT('Ctrl Pts',(-47.7414452899411,-26.1688071749961,
177.206816180124));
#14534=CARTESIAN_POINT('Ctrl Pts',(-47.2997616792461,-25.8707230428421,
176.259912393579));
#14535=CARTESIAN_POINT('Ctrl Pts',(-47.3254088075791,-25.7696878441865,
175.668385446485));
#14536=CARTESIAN_POINT('Ctrl Pts',(-47.8755348089008,-25.6608852645148,
174.730075629747));
#14537=CARTESIAN_POINT('Ctrl Pts',(-48.3883745667453,-25.6533154874374,
174.409130171609));
#14538=CARTESIAN_POINT('Ctrl Pts',(-49.4697935970405,-25.6493947609597,
174.331547147859));
#14539=CARTESIAN_POINT('Ctrl Pts',(-50.0242338430418,-25.649381701477,174.571983854445));
#14540=CARTESIAN_POINT('Ctrl Pts',(-50.7048786270563,-25.5680766842178,
175.408205503607));
#14541=CARTESIAN_POINT('Ctrl Pts',(-50.8241348799264,-25.4835527568238,
175.999504945815));
#14542=CARTESIAN_POINT('Ctrl Pts',(-50.5299373615978,-25.2151761375736,
177.003363164347));
#14543=CARTESIAN_POINT('Ctrl Pts',(-50.1239438073276,-25.0297634587285,
177.413176265946));
#14544=CARTESIAN_POINT('Ctrl Pts',(-49.1505246752548,-24.6280758402134,
177.688626402201));
#14545=CARTESIAN_POINT('Ctrl Pts',(-48.5986534337901,-24.4145815428545,
177.549736774231));
#14546=CARTESIAN_POINT('Ctrl Pts',(-47.8611459428243,-24.0600384609719,
176.839550282587));
#14547=CARTESIAN_POINT('Ctrl Pts',(-47.6799485846058,-23.9185188665616,
176.282427966132));
#14548=CARTESIAN_POINT('Ctrl Pts',(-47.8667875018081,-23.7413010936383,
175.228664295839));
#14549=CARTESIAN_POINT('Ctrl Pts',(-48.2335406641398,-23.7053609783786,
174.748651320702));
#14550=CARTESIAN_POINT('Ctrl Pts',(-49.2178139490401,-23.6827183215843,
174.294936194443));
#14551=CARTESIAN_POINT('Ctrl Pts',(-49.8219962257384,-23.6923479099038,
174.323992647469));
#14552=CARTESIAN_POINT('Ctrl Pts',(-50.7591498572879,-23.6591435932359,
174.876124371948));
#14553=CARTESIAN_POINT('Ctrl Pts',(-51.077522753783,-23.6134950148359,175.39172485521));
#14554=CARTESIAN_POINT('Ctrl Pts',(-51.1535820381579,-23.415693423287,176.455061557909));
#14555=CARTESIAN_POINT('Ctrl Pts',(-50.918643706726,-23.2638702537623,176.988610346676));
#14556=CARTESIAN_POINT('Ctrl Pts',(-50.1109113395739,-22.8948872174005,
177.611393006538));
#14557=CARTESIAN_POINT('Ctrl Pts',(-49.550353441179,-22.680074585543,177.689808241912));
#14558=CARTESIAN_POINT('Ctrl Pts',(-48.6137447048011,-22.28702457331,177.311258226648));
#14559=CARTESIAN_POINT('Ctrl Pts',(-48.2490117887893,-22.1098470443037,
176.862573175931));
#14560=CARTESIAN_POINT('Ctrl Pts',(-48.0569364843034,-21.8588516971627,
175.821098220226));
#14561=CARTESIAN_POINT('Ctrl Pts',(-48.2348449020816,-21.7860567828884,
175.244332219005));
#14562=CARTESIAN_POINT('Ctrl Pts',(-49.0386897150743,-21.7181941257994,
174.442583421401));
#14563=CARTESIAN_POINT('Ctrl Pts',(-49.6927278496366,-21.7268807239962,
174.267611662058));
#14564=CARTESIAN_POINT('Ctrl Pts',(-50.8411043798997,-21.7141199241716,
174.588524908528));
#14565=CARTESIAN_POINT('Ctrl Pts',(-51.3094013702521,-21.6876269507243,
175.077312328235));
#14566=CARTESIAN_POINT('Ctrl Pts',(-51.5921855585383,-21.5071481278118,
176.224756535618));
#14567=CARTESIAN_POINT('Ctrl Pts',(-51.3974806497779,-21.3525654190584,
176.857134695111));
#14568=CARTESIAN_POINT('Ctrl Pts',(-50.5541169969121,-20.9549536496367,
177.606432421015));
#14569=CARTESIAN_POINT('Ctrl Pts',(-49.9226700094089,-20.7151144402318,
177.707627413831));
#14570=CARTESIAN_POINT('Ctrl Pts',(-48.9071810235129,-20.2857229365746,
177.254800594979));
#14571=CARTESIAN_POINT('Ctrl Pts',(-48.539258060867,-20.0973264562627,176.718436772752));
#14572=CARTESIAN_POINT('Ctrl Pts',(-48.475069365768,-19.8507243142978,175.553477519371));
#14573=CARTESIAN_POINT('Ctrl Pts',(-48.7817617425817,-19.793065331538,174.952184411851));
#14574=CARTESIAN_POINT('Ctrl Pts',(-49.7883433018784,-19.7521647995451,
174.308551222089));
#14575=CARTESIAN_POINT('Ctrl Pts',(-50.4672686416896,-19.7660480884512,
174.284275257332));
#14576=CARTESIAN_POINT('Ctrl Pts',(-51.5185621567429,-19.7338211938064,
174.853733695028));
#14577=CARTESIAN_POINT('Ctrl Pts',(-51.8704305933054,-19.6836035315617,
175.436932234299));
#14578=CARTESIAN_POINT('Ctrl Pts',(-51.8843323266907,-19.4527281797322,
176.606134032902));
#14579=CARTESIAN_POINT('Ctrl Pts',(-51.5571193795133,-19.2721887380014,
177.170821269618));
#14580=CARTESIAN_POINT('Ctrl Pts',(-50.5738822832083,-18.8483164964054,
177.696322750616));
#14581=CARTESIAN_POINT('Ctrl Pts',(-49.9420101663495,-18.6096692642048,
177.644259926591));
#14582=CARTESIAN_POINT('Ctrl Pts',(-49.0472024681392,-18.2021277928874,
176.964465534643));
#14583=CARTESIAN_POINT('Ctrl Pts',(-48.8080140865945,-18.0389468515475,
176.349664596734));
#14584=CARTESIAN_POINT('Ctrl Pts',(-49.0066488397389,-17.8423059144124,
175.186793179499));
#14585=CARTESIAN_POINT('Ctrl Pts',(-49.4421820059815,-17.8082452535064,
174.661978305101));
#14586=CARTESIAN_POINT('Ctrl Pts',(-50.56604357313,-17.7913894148755,174.265152819574));
#14587=CARTESIAN_POINT('Ctrl Pts',(-51.2311395254822,-17.8022399917982,
174.391161445375));
#14588=CARTESIAN_POINT('Ctrl Pts',(-52.1286453083844,-17.7409968363402,
175.174698745784));
#14589=CARTESIAN_POINT('Ctrl Pts',(-52.340061283037,-17.6649540872478,175.813880719354));
#14590=CARTESIAN_POINT('Ctrl Pts',(-52.1027685307223,-17.384247754716,176.951110854015));
#14591=CARTESIAN_POINT('Ctrl Pts',(-51.6569691297711,-17.1812314095055,
177.42208876923));
#14592=CARTESIAN_POINT('Ctrl Pts',(-50.5803007618318,-16.7386138153048,
177.697510231007));
#14593=CARTESIAN_POINT('Ctrl Pts',(-49.9722430688612,-16.5033958825231,
177.495874655633));
#14594=CARTESIAN_POINT('Ctrl Pts',(-49.2598451033921,-16.1323520825764,
176.614580397518));
#14595=CARTESIAN_POINT('Ctrl Pts',(-49.1633964478354,-15.9963838869222,
175.958557394859));
#14596=CARTESIAN_POINT('Ctrl Pts',(-49.6135825845651,-15.8488720097956,
174.863627023648));
#14597=CARTESIAN_POINT('Ctrl Pts',(-50.1513088289339,-15.8357216637453,
174.451396860398));
#14598=CARTESIAN_POINT('Ctrl Pts',(-51.3373123393945,-15.8295083514664,
174.304991255183));
#14599=CARTESIAN_POINT('Ctrl Pts',(-51.9598057434752,-15.8324905082382,
174.577589691682));
#14600=CARTESIAN_POINT('Ctrl Pts',(-52.662356604517,-15.7329936013494,175.540542955831));
#14601=CARTESIAN_POINT('Ctrl Pts',(-52.7287365437827,-15.6278770852026,
176.211335092655));
#14602=CARTESIAN_POINT('Ctrl Pts',(-52.2404503570114,-15.2999892249187,
177.248966419092));
#14603=CARTESIAN_POINT('Ctrl Pts',(-51.7049290320028,-15.079336195701,177.599407337456));
#14604=CARTESIAN_POINT('Ctrl Pts',(-50.599341197491,-14.6318604318474,177.611289749054));
#14605=CARTESIAN_POINT('Ctrl Pts',(-50.0563698831837,-14.4102803084529,
177.271399907022));
#14606=CARTESIAN_POINT('Ctrl Pts',(-49.5511866458666,-14.0779293284932,
176.24060069501));
#14607=CARTESIAN_POINT('Ctrl Pts',(-49.604058679892,-13.971112568136,175.571774049481));
#14608=CARTESIAN_POINT('Ctrl Pts',(-50.2895824050587,-13.8682646399117,
174.596554366676));
#14609=CARTESIAN_POINT('Ctrl Pts',(-50.9089033822508,-13.8698152300494,
174.310925422501));
#14610=CARTESIAN_POINT('Ctrl Pts',(-52.0945937584551,-13.8647732522077,
174.438441317441));
#14611=CARTESIAN_POINT('Ctrl Pts',(-52.6396705452532,-13.8524570813917,
174.840092836798));
#14612=CARTESIAN_POINT('Ctrl Pts',(-53.1114861845869,-13.7091720746061,
175.926135983292));
#14613=CARTESIAN_POINT('Ctrl Pts',(-53.0273981908184,-13.5760746720968,
176.585468457757));
#14614=CARTESIAN_POINT('Ctrl Pts',(-52.3273047331872,-13.2061141571923,
177.480731662196));
#14615=CARTESIAN_POINT('Ctrl Pts',(-51.7260689896615,-12.9732036309654,
177.694033962224));
#14616=CARTESIAN_POINT('Ctrl Pts',(-50.6444965881338,-12.5296009109336,
177.439340266607));
#14617=CARTESIAN_POINT('Ctrl Pts',(-50.1880101288259,-12.323622761024,176.975929902189));
#14618=CARTESIAN_POINT('Ctrl Pts',(-49.9332603826239,-12.0409453485109,
175.846473225312));
#14619=CARTESIAN_POINT('Ctrl Pts',(-50.1325085529845,-11.9618298866148,
175.20357102314));
#14620=CARTESIAN_POINT('Ctrl Pts',(-51.0139495749547,-11.8975707104174,
174.402850839007));
#14621=CARTESIAN_POINT('Ctrl Pts',(-51.6770380739026,-11.9086053392238,
174.263669429449));
#14622=CARTESIAN_POINT('Ctrl Pts',(-52.8102442474793,-11.89211453585,174.644220443453));
#14623=CARTESIAN_POINT('Ctrl Pts',(-53.2534129688289,-11.860550625243,175.158200214442));
#14624=CARTESIAN_POINT('Ctrl Pts',(-53.4727724514858,-11.667970777174,176.317676214963));
#14625=CARTESIAN_POINT('Ctrl Pts',(-53.2447122957938,-11.5059876351892,
176.940267405791));
#14626=CARTESIAN_POINT('Ctrl Pts',(-52.3630606041574,-11.1023742765951,
177.633671542876));
#14627=CARTESIAN_POINT('Ctrl Pts',(-51.7328063873735,-10.863413150139,177.698996091772));
#14628=CARTESIAN_POINT('Ctrl Pts',(-50.7387975664535,-10.4373493069837,
177.194617067458));
#14629=CARTESIAN_POINT('Ctrl Pts',(-50.4003959556136,-10.2552411513015,
176.636362249629));
#14630=CARTESIAN_POINT('Ctrl Pts',(-50.3964887911414,-10.0195709762704,
175.464836254896));
#14631=CARTESIAN_POINT('Ctrl Pts',(-50.7352645697859,-9.96785241001128,
174.878086269107));
#14632=CARTESIAN_POINT('Ctrl Pts',(-51.7761584941716,-9.93363014738946,
174.290073576044));
#14633=CARTESIAN_POINT('Ctrl Pts',(-52.4578743221659,-9.94721824196466,
174.301034748671));
#14634=CARTESIAN_POINT('Ctrl Pts',(-53.4723487166264,-9.90911175935534,
174.927224952557));
#14635=CARTESIAN_POINT('Ctrl Pts',(-53.7905639694071,-9.85304000489839,
175.522456262626));
#14636=CARTESIAN_POINT('Ctrl Pts',(-53.7495974866252,-9.61086987508902,
176.689642787431));
#14637=CARTESIAN_POINT('Ctrl Pts',(-53.3913473444599,-9.42486391207369,
177.234457154129));
#14638=CARTESIAN_POINT('Ctrl Pts',(-52.3804909291071,-8.9950096827268,177.705080880716));
#14639=CARTESIAN_POINT('Ctrl Pts',(-51.7506169575959,-8.75656955580448,
177.617528508224));
#14640=CARTESIAN_POINT('Ctrl Pts',(-50.8938217209944,-8.35631416012115,
176.884644400558));
#14641=CARTESIAN_POINT('Ctrl Pts',(-50.686386739593,-8.19840449522365,176.254364811283));
#14642=CARTESIAN_POINT('Ctrl Pts',(-50.9496816541175,-8.01563271032117,
175.10646784668));
#14643=CARTESIAN_POINT('Ctrl Pts',(-51.4086597834924,-7.98657238824085,
174.608429324338));
#14644=CARTESIAN_POINT('Ctrl Pts',(-52.5506583028891,-7.97253715897243,
174.264721414109));
#14645=CARTESIAN_POINT('Ctrl Pts',(-53.2085070979977,-7.98255305121696,
174.427141629608));
#14646=CARTESIAN_POINT('Ctrl Pts',(-54.0661826067832,-7.91293346685192,
175.257046778597));
#14647=CARTESIAN_POINT('Ctrl Pts',(-54.2443196068901,-7.83026930904402,
175.907383805075));
#14648=CARTESIAN_POINT('Ctrl Pts',(-53.9449265679421,-7.53766373675317,
177.027297077911));
#14649=CARTESIAN_POINT('Ctrl Pts',(-53.4737144264175,-7.32885697968307,
177.474235384447));
#14650=CARTESIAN_POINT('Ctrl Pts',(-52.3866301268079,-6.88556912331281,
177.682767568372));
#14651=CARTESIAN_POINT('Ctrl Pts',(-51.7946034524202,-6.6539762900198,177.44919290535));
#14652=CARTESIAN_POINT('Ctrl Pts',(-51.1242376556131,-6.29031677842802,
176.53135144958));
#14653=CARTESIAN_POINT('Ctrl Pts',(-51.0636455015902,-6.16179111781231,
175.868699032101));
#14654=CARTESIAN_POINT('Ctrl Pts',(-51.5708785507503,-6.02461835391231,
174.795021951807));
#14655=CARTESIAN_POINT('Ctrl Pts',(-52.1305414737447,-6.01557067494389,
174.410384417273));
#14656=CARTESIAN_POINT('Ctrl Pts',(-53.3239707675344,-6.01072022664985,
174.329110015938));
#14657=CARTESIAN_POINT('Ctrl Pts',(-53.9334177584311,-6.01040522494539,
174.634606029695));
#14658=CARTESIAN_POINT('Ctrl Pts',(-54.5783977308191,-5.90111793801205,
175.631553651875));
#14659=CARTESIAN_POINT('Ctrl Pts',(-54.6093650217473,-5.78956533803437,
176.299320421659));
#14660=CARTESIAN_POINT('Ctrl Pts',(-54.0728671794864,-5.45185644429227,
177.309544041851));
#14661=CARTESIAN_POINT('Ctrl Pts',(-53.5182109168208,-5.22801082267814,
177.628618080665));
#14662=CARTESIAN_POINT('Ctrl Pts',(-52.4111095558568,-4.77949537513279,
177.578747218087));
#14663=CARTESIAN_POINT('Ctrl Pts',(-51.8857104064777,-4.56119881916171,
177.207895099161));
#14664=CARTESIAN_POINT('Ctrl Pts',(-51.4375681932236,-4.23993965724606,
176.147216345704));
#14665=CARTESIAN_POINT('Ctrl Pts',(-51.5255341013567,-4.13891120462634,
175.478088476179));
#14666=CARTESIAN_POINT('Ctrl Pts',(-52.2621121714531,-4.04739311840896,
174.545543255356));
#14667=CARTESIAN_POINT('Ctrl Pts',(-52.8911810801,-4.05123090724587,174.294043710706));
#14668=CARTESIAN_POINT('Ctrl Pts',(-54.0705541410016,-4.04422766004653,
174.477498952297));
#14669=CARTESIAN_POINT('Ctrl Pts',(-54.593284417315,-4.02816934534973,174.908686002258));
#14670=CARTESIAN_POINT('Ctrl Pts',(-55.0092587601974,-3.87346271742067,
176.018250487428));
#14671=CARTESIAN_POINT('Ctrl Pts',(-54.8907029615328,-3.73358556412494,
176.67236673678));
#14672=CARTESIAN_POINT('Ctrl Pts',(-54.1422797098421,-3.35431610458726,
177.524634651606));
#14673=CARTESIAN_POINT('Ctrl Pts',(-53.5287781394068,-3.11818277146878,
177.704881014433));
#14674=CARTESIAN_POINT('Ctrl Pts',(-52.4666030700143,-2.67965003658039,
177.385814188219));
#14675=CARTESIAN_POINT('Ctrl Pts',(-52.037952109723,-2.47949238143003,176.900644117435));
#14676=CARTESIAN_POINT('Ctrl Pts',(-51.8369606432704,-2.20643344946428,
175.75693673757));
#14677=CARTESIAN_POINT('Ctrl Pts',(-52.0709636415419,-2.13467360272607,
175.124746251973));
#14678=CARTESIAN_POINT('Ctrl Pts',(-52.9948906247979,-2.07782438513344,
174.368185237747));
#14679=CARTESIAN_POINT('Ctrl Pts',(-53.6658603596095,-2.09023021076396,
174.26394539811));
#14680=CARTESIAN_POINT('Ctrl Pts',(-54.7763899734937,-2.0695796979931,174.705748499134));
#14681=CARTESIAN_POINT('Ctrl Pts',(-55.193636646253,-2.03216929631525,175.243747077929));
#14682=CARTESIAN_POINT('Ctrl Pts',(-55.2990804121262,-1.89289436927212,
176.038719570758));
#14683=CARTESIAN_POINT('Ctrl Pts',(-55.2875271080061,-1.8476232285876,176.255654667139));
#14684=CARTESIAN_POINT('Ctrl Pts',(-55.2062064365128,-1.76817883590891,
176.561034862255));
#14685=CARTESIAN_POINT('Ctrl Pts',(-55.1692797902087,-1.73965218400568,
176.660101738528));
#14686=CARTESIAN_POINT('Ctrl Pts',(-55.100781391479,-1.69439363416682,176.801019080259));
#14687=CARTESIAN_POINT('Ctrl Pts',(-55.0757487692566,-1.67889591755103,
176.846705834293));
#14688=CARTESIAN_POINT('Ctrl Pts',(-55.0215162671022,-1.64716827604208,
176.934897450488));
#14689=CARTESIAN_POINT('Ctrl Pts',(-54.9831012773678,-1.62642361195712,
176.988063802692));
#14690=CARTESIAN_POINT('Ctrl Pts',(-54.9611536226478,-1.61438316700751,
177.018013216499));
#14691=CARTESIAN_POINT('Ctrl Pts',(-49.4509304485228,-27.5317240793367,
176.63793339336));
#14692=CARTESIAN_POINT('Ctrl Pts',(-49.4291393884885,-27.5076562767722,
176.671636728953));
#14693=CARTESIAN_POINT('Ctrl Pts',(-49.4023252814003,-27.49622653535,176.696313164424));
#14694=CARTESIAN_POINT('Ctrl Pts',(-49.3476504462613,-27.4590129437169,
176.750465273433));
#14695=CARTESIAN_POINT('Ctrl Pts',(-49.3184236390985,-27.4399206811032,
176.775937697594));
#14696=CARTESIAN_POINT('Ctrl Pts',(-49.2266057058354,-27.3820561699738,
176.84602259684));
#14697=CARTESIAN_POINT('Ctrl Pts',(-49.1608892759397,-27.3435420466437,
176.883532818161));
#14698=CARTESIAN_POINT('Ctrl Pts',(-48.9520433277106,-27.2233369569446,
176.969216598557));
#14699=CARTESIAN_POINT('Ctrl Pts',(-48.7994772773074,-27.140753695473,176.988359561004));
#14700=CARTESIAN_POINT('Ctrl Pts',(-48.3519200751284,-26.8936813947759,
176.923562975379));
#14701=CARTESIAN_POINT('Ctrl Pts',(-48.0823456895327,-26.734263465041,176.708580257885));
#14702=CARTESIAN_POINT('Ctrl Pts',(-47.8449430900585,-26.4783672905687,
176.126725989992));
#14703=CARTESIAN_POINT('Ctrl Pts',(-47.8767939676907,-26.3778568396964,
175.764012928805));
#14704=CARTESIAN_POINT('Ctrl Pts',(-48.2463197375522,-26.2327937589041,
175.197492946021));
#14705=CARTESIAN_POINT('Ctrl Pts',(-48.5747178643875,-26.1889682126354,
175.01137731386));
#14706=CARTESIAN_POINT('Ctrl Pts',(-49.2462054467177,-26.1087803247027,
174.981703215741));
#14707=CARTESIAN_POINT('Ctrl Pts',(-49.5907543357586,-26.0676212071441,
175.137035562833));
#14708=CARTESIAN_POINT('Ctrl Pts',(-50.009388927793,-25.9343746307825,175.661646016755));
#14709=CARTESIAN_POINT('Ctrl Pts',(-50.0783027352647,-25.8394975457309,
176.025761110018));
#14710=CARTESIAN_POINT('Ctrl Pts',(-49.8988780633176,-25.5959204367964,
176.628597112503));
#14711=CARTESIAN_POINT('Ctrl Pts',(-49.6518990744916,-25.4405710050954,
176.873652740602));
#14712=CARTESIAN_POINT('Ctrl Pts',(-49.0655102948359,-25.1120926941016,
177.024416386827));
#14713=CARTESIAN_POINT('Ctrl Pts',(-48.7382306499136,-24.9412172473198,
176.927283980104));
#14714=CARTESIAN_POINT('Ctrl Pts',(-48.31783324883,-24.6506072191097,176.48408449858));
#14715=CARTESIAN_POINT('Ctrl Pts',(-48.2223197693695,-24.5249427903147,
176.139359044285));
#14716=CARTESIAN_POINT('Ctrl Pts',(-48.3708320195333,-24.3389138358785,
175.495466335841));
#14717=CARTESIAN_POINT('Ctrl Pts',(-48.6129161956615,-24.2782922597527,
175.208867671322));
#14718=CARTESIAN_POINT('Ctrl Pts',(-49.2318343995499,-24.18785243492,174.949625492768));
#14719=CARTESIAN_POINT('Ctrl Pts',(-49.6097264895464,-24.153250081799,174.976039603467));
#14720=CARTESIAN_POINT('Ctrl Pts',(-50.1907740657023,-24.0499499019578,
175.330958269522));
#14721=CARTESIAN_POINT('Ctrl Pts',(-50.3830787723347,-23.9792981329734,
175.653008106489));
#14722=CARTESIAN_POINT('Ctrl Pts',(-50.427159666228,-23.7781136900229,176.297852422263));
#14723=CARTESIAN_POINT('Ctrl Pts',(-50.2832787288339,-23.643180828803,176.621446326487));
#14724=CARTESIAN_POINT('Ctrl Pts',(-49.7924641893585,-23.3338917128074,
176.988303084673));
#14725=CARTESIAN_POINT('Ctrl Pts',(-49.455479895244,-23.1615506277796,177.024112028042));
#14726=CARTESIAN_POINT('Ctrl Pts',(-48.9089639726264,-22.8463871647641,
176.778406765063));
#14727=CARTESIAN_POINT('Ctrl Pts',(-48.699448601228,-22.6985448431478,176.497595410894));
#14728=CARTESIAN_POINT('Ctrl Pts',(-48.6153144001997,-22.4669397150842,
175.854418703293));
#14729=CARTESIAN_POINT('Ctrl Pts',(-48.7438560906085,-22.3839338201049,
175.504557803726));
#14730=CARTESIAN_POINT('Ctrl Pts',(-49.2595227997445,-22.2634194140522,
175.031489327737));
#14731=CARTESIAN_POINT('Ctrl Pts',(-49.6731287428438,-22.2242903845664,
174.93387435438));
#14732=CARTESIAN_POINT('Ctrl Pts',(-50.3871280758708,-22.1273049999089,
175.149675576275));
#14733=CARTESIAN_POINT('Ctrl Pts',(-50.6724659987737,-22.0667095289654,
175.454257853488));
#14734=CARTESIAN_POINT('Ctrl Pts',(-50.8432291330538,-21.8630647724227,
176.162580877915));
#14735=CARTESIAN_POINT('Ctrl Pts',(-50.7223573298116,-21.7238000115757,
176.543315008655));
#14736=CARTESIAN_POINT('Ctrl Pts',(-50.2109398093855,-21.3899066275767,
176.985840165295));
#14737=CARTESIAN_POINT('Ctrl Pts',(-49.8297406934723,-21.1967740899633,
177.034608068765));
#14738=CARTESIAN_POINT('Ctrl Pts',(-49.2383022679982,-20.8522162432738,
176.742643808163));
#14739=CARTESIAN_POINT('Ctrl Pts',(-49.0288695410029,-20.692930608689,176.406589078903));
#14740=CARTESIAN_POINT('Ctrl Pts',(-49.026421127215,-20.4577766282769,175.692082743004));
#14741=CARTESIAN_POINT('Ctrl Pts',(-49.2307435857662,-20.3815547180372,
175.331094438645));
#14742=CARTESIAN_POINT('Ctrl Pts',(-49.8766835352141,-20.269544445424,174.953525304613));
#14743=CARTESIAN_POINT('Ctrl Pts',(-50.2982947167721,-20.234888952096,174.950394529643));
#14744=CARTESIAN_POINT('Ctrl Pts',(-50.9484787003876,-20.125016744292,175.316388781725));
#14745=CARTESIAN_POINT('Ctrl Pts',(-51.1618775184403,-20.046547250015,175.681463428659));
#14746=CARTESIAN_POINT('Ctrl Pts',(-51.1680956128,-19.8172503157992,176.389348367045));
#14747=CARTESIAN_POINT('Ctrl Pts',(-50.9669054157941,-19.6595598406301,
176.731136037536));
#14748=CARTESIAN_POINT('Ctrl Pts',(-50.3735191706099,-19.3104097045359,
177.03446439702));
#14749=CARTESIAN_POINT('Ctrl Pts',(-49.9983681415115,-19.122445314997,176.992069263085));
#14750=CARTESIAN_POINT('Ctrl Pts',(-49.4783291859613,-18.7856098039383,
176.558083132201));
#14751=CARTESIAN_POINT('Ctrl Pts',(-49.3516920035876,-18.6452157185327,
176.179591346513));
#14752=CARTESIAN_POINT('Ctrl Pts',(-49.5099669630901,-18.4404938180664,
175.471248155379));
#14753=CARTESIAN_POINT('Ctrl Pts',(-49.7966826107081,-18.3761869903911,
175.157298861455));
#14754=CARTESIAN_POINT('Ctrl Pts',(-50.5005002255267,-18.2813908051205,
174.934848239897));
#14755=CARTESIAN_POINT('Ctrl Pts',(-50.9163195448478,-18.2427172185017,
175.022527695559));
#14756=CARTESIAN_POINT('Ctrl Pts',(-51.4689900750814,-18.1145211614547,
175.516882458909));
#14757=CARTESIAN_POINT('Ctrl Pts',(-51.5957313663424,-18.0233261232984,
175.908710828391));
#14758=CARTESIAN_POINT('Ctrl Pts',(-51.4475718943418,-17.7582443007608,
176.601404917962));
#14759=CARTESIAN_POINT('Ctrl Pts',(-51.1767645681398,-17.5900571721881,
176.879541091562));
#14760=CARTESIAN_POINT('Ctrl Pts',(-50.5307383316194,-17.2301836239675,
177.028185493998));
#14761=CARTESIAN_POINT('Ctrl Pts',(-50.1698955770676,-17.0410908031352,
176.891376748831));
#14762=CARTESIAN_POINT('Ctrl Pts',(-49.7689671613288,-16.733171977968,176.344861065041));
#14763=CARTESIAN_POINT('Ctrl Pts',(-49.7283236820348,-16.606509721343,175.939499115166));
#14764=CARTESIAN_POINT('Ctrl Pts',(-50.039329025483,-16.4317046321664,175.276913396961));
#14765=CARTESIAN_POINT('Ctrl Pts',(-50.3811663065111,-16.3819545297351,
175.034692629757));
#14766=CARTESIAN_POINT('Ctrl Pts',(-51.1285550225506,-16.289595439286,174.965429755586));
#14767=CARTESIAN_POINT('Ctrl Pts',(-51.5107791504261,-16.247329788901,175.141829956289));
#14768=CARTESIAN_POINT('Ctrl Pts',(-51.9410271179475,-16.0950193648309,
175.742297045045));
#14769=CARTESIAN_POINT('Ctrl Pts',(-51.9772772372669,-15.9825461483302,
176.155328152494));
#14770=CARTESIAN_POINT('Ctrl Pts',(-51.6813604170028,-15.6948169276305,
176.775145838897));
#14771=CARTESIAN_POINT('Ctrl Pts',(-51.3553093740791,-15.5131006527082,
176.981869312707));
#14772=CARTESIAN_POINT('Ctrl Pts',(-50.6958293220101,-15.1512003838696,
176.968860943967));
#14773=CARTESIAN_POINT('Ctrl Pts',(-50.3793004471536,-14.974461104635,176.752883253889));
#14774=CARTESIAN_POINT('Ctrl Pts',(-50.1044053585231,-14.6849545931669,
176.110550614429));
#14775=CARTESIAN_POINT('Ctrl Pts',(-50.1562892256051,-14.5790344049375,
175.704381183727));
#14776=CARTESIAN_POINT('Ctrl Pts',(-50.6091148636379,-14.4310075872896,
175.119365593043));
#14777=CARTESIAN_POINT('Ctrl Pts',(-51.0040002342342,-14.3877335732316,
174.956144468714));
#14778=CARTESIAN_POINT('Ctrl Pts',(-51.7368765161625,-14.2984333198446,
175.052400920313));
#14779=CARTESIAN_POINT('Ctrl Pts',(-52.0746787278137,-14.2446881736679,
175.307721150405));
#14780=CARTESIAN_POINT('Ctrl Pts',(-52.3618029222314,-14.0653384618121,
175.979593696432));
#14781=CARTESIAN_POINT('Ctrl Pts',(-52.3085224478133,-13.9393545956389,
176.378830696363));
#14782=CARTESIAN_POINT('Ctrl Pts',(-51.8806097785072,-13.6203167705008,
176.914733769747));
#14783=CARTESIAN_POINT('Ctrl Pts',(-51.5196766160896,-13.4348339691437,
177.033422941425));
#14784=CARTESIAN_POINT('Ctrl Pts',(-50.8796650354229,-13.0760747213028,
176.857816848924));
#14785=CARTESIAN_POINT('Ctrl Pts',(-50.6171262914928,-12.905954023484,176.563294278628));
#14786=CARTESIAN_POINT('Ctrl Pts',(-50.4974416512911,-12.6523824704848,
175.874038771655));
#14787=CARTESIAN_POINT('Ctrl Pts',(-50.6384867622314,-12.5605842376971,
175.481424733232));
#14788=CARTESIAN_POINT('Ctrl Pts',(-51.2082627201524,-12.4357774521296,
175.006422958104));
#14789=CARTESIAN_POINT('Ctrl Pts',(-51.6220204445227,-12.3999030775176,
174.932310130414));
#14790=CARTESIAN_POINT('Ctrl Pts',(-52.3278760969134,-12.2994377602634,
175.185413156184));
#14791=CARTESIAN_POINT('Ctrl Pts',(-52.5969267492371,-12.2353856775628,
175.505423112887));
#14792=CARTESIAN_POINT('Ctrl Pts',(-52.7283564524999,-12.0255423744405,
176.2175433277));
#14793=CARTESIAN_POINT('Ctrl Pts',(-52.5846730379872,-11.8782873041682,
176.594912064781));
#14794=CARTESIAN_POINT('Ctrl Pts',(-52.0559417647627,-11.5457913524836,
176.999632681105));
#14795=CARTESIAN_POINT('Ctrl Pts',(-51.6759748702359,-11.3536364027873,
177.029489895259));
#14796=CARTESIAN_POINT('Ctrl Pts',(-51.0935427887116,-11.0064931497742,
176.702663500826));
#14797=CARTESIAN_POINT('Ctrl Pts',(-50.9048767955961,-10.8544314216914,
176.357244031546));
#14798=CARTESIAN_POINT('Ctrl Pts',(-50.9399834898308,-10.6247204655602,
175.63759182164));
#14799=CARTESIAN_POINT('Ctrl Pts',(-51.1643267174014,-10.5520247194105,
175.286394351447));
#14800=CARTESIAN_POINT('Ctrl Pts',(-51.827873009513,-10.4447251212865,174.944424130566));
#14801=CARTESIAN_POINT('Ctrl Pts',(-52.2552179028772,-10.4077182802165,
174.964702471846));
#14802=CARTESIAN_POINT('Ctrl Pts',(-52.8763669051787,-10.2968258721765,
175.360239151239));
#14803=CARTESIAN_POINT('Ctrl Pts',(-53.071683414474,-10.215593033151,175.73103698433));
#14804=CARTESIAN_POINT('Ctrl Pts',(-53.0437675059112,-9.97549498249197,
176.443487491333));
#14805=CARTESIAN_POINT('Ctrl Pts',(-52.825568431635,-9.81766629245078,176.768582048511));
#14806=CARTESIAN_POINT('Ctrl Pts',(-52.2143534856381,-9.46331409552581,
177.038351228206));
#14807=CARTESIAN_POINT('Ctrl Pts',(-51.8411412849432,-9.27545967967225,
176.973585868646));
#14808=CARTESIAN_POINT('Ctrl Pts',(-51.3467118649778,-8.94477024831946,
176.509526159241));
#14809=CARTESIAN_POINT('Ctrl Pts',(-51.2404836863797,-8.80483732687828,
176.117599105019));
#14810=CARTESIAN_POINT('Ctrl Pts',(-51.4349583516297,-8.61185430488912,
175.425788146171));
#14811=CARTESIAN_POINT('Ctrl Pts',(-51.7335486000159,-8.55040314694308,
175.126384517701));
#14812=CARTESIAN_POINT('Ctrl Pts',(-52.4549196826756,-8.45481293341497,
174.935526629257));
#14813=CARTESIAN_POINT('Ctrl Pts',(-52.8607223331575,-8.41739346719437,
175.04474867484));
#14814=CARTESIAN_POINT('Ctrl Pts',(-53.3897252776085,-8.28282809274167,
175.568595073035));
#14815=CARTESIAN_POINT('Ctrl Pts',(-53.4952826969923,-8.1872595086965,175.966830212787));
#14816=CARTESIAN_POINT('Ctrl Pts',(-53.3101642867802,-7.91637813164073,
176.645610777581));
#14817=CARTESIAN_POINT('Ctrl Pts',(-53.02056762136,-7.74105352934409,176.910070201754));
#14818=CARTESIAN_POINT('Ctrl Pts',(-52.3751524190461,-7.38599804306437,
177.017607675131));
#14819=CARTESIAN_POINT('Ctrl Pts',(-52.0232566558232,-7.19924964083975,
176.864225220861));
#14820=CARTESIAN_POINT('Ctrl Pts',(-51.6458284953554,-6.89163712519652,
176.29020971736));
#14821=CARTESIAN_POINT('Ctrl Pts',(-51.6277644578821,-6.7724816775637,175.885858382765));
#14822=CARTESIAN_POINT('Ctrl Pts',(-51.9747906942483,-6.6028499237395,175.235443151034));
#14823=CARTESIAN_POINT('Ctrl Pts',(-52.3299962525585,-6.55546850196264,
175.011060208135));
#14824=CARTESIAN_POINT('Ctrl Pts',(-53.0782096175287,-6.46444741567071,
174.9816560919));
#14825=CARTESIAN_POINT('Ctrl Pts',(-53.4553178435249,-6.41778988524295,
175.181401713961));
#14826=CARTESIAN_POINT('Ctrl Pts',(-53.8466529433518,-6.26265155715774,
175.795420851333));
#14827=CARTESIAN_POINT('Ctrl Pts',(-53.864188958285,-6.14704492720176,176.206287912404));
#14828=CARTESIAN_POINT('Ctrl Pts',(-53.5358416511927,-5.84903598495515,
176.813977641948));
#14829=CARTESIAN_POINT('Ctrl Pts',(-53.2017653978813,-5.66889429660941,
176.99856451113));
#14830=CARTESIAN_POINT('Ctrl Pts',(-52.5405403606902,-5.30479587533914,
176.947248559284));
#14831=CARTESIAN_POINT('Ctrl Pts',(-52.2356929075399,-5.13012364220884,
176.712058308829));
#14832=CARTESIAN_POINT('Ctrl Pts',(-51.9967219623743,-4.84888631606004,
176.054758979681));
#14833=CARTESIAN_POINT('Ctrl Pts',(-52.0727509238964,-4.74401755802611,
175.645031481929));
#14834=CARTESIAN_POINT('Ctrl Pts',(-52.5505176724514,-4.6056507589775,175.091566392661));
#14835=CARTESIAN_POINT('Ctrl Pts',(-52.9499574883172,-4.56374410570602,
174.946492448473));
#14836=CARTESIAN_POINT('Ctrl Pts',(-53.685231908784,-4.47066113931358,175.078743542747));
#14837=CARTESIAN_POINT('Ctrl Pts',(-54.0046084640979,-4.41655583760205,
175.349203817777));
#14838=CARTESIAN_POINT('Ctrl Pts',(-54.2577428662421,-4.2288827567675,176.036685454146));
#14839=CARTESIAN_POINT('Ctrl Pts',(-54.1828214302285,-4.09851492101137,
176.431966849275));
#14840=CARTESIAN_POINT('Ctrl Pts',(-53.7276699197103,-3.77548143923658,
176.939160233154));
#14841=CARTESIAN_POINT('Ctrl Pts',(-53.3559275609679,-3.58443131799679,
177.036850521868));
#14842=CARTESIAN_POINT('Ctrl Pts',(-52.7340684542075,-3.23387064793483,
176.825149499914));
#14843=CARTESIAN_POINT('Ctrl Pts',(-52.4865052787647,-3.06716804391598,
176.519600526728));
#14844=CARTESIAN_POINT('Ctrl Pts',(-52.4000162427049,-2.81575249291398,
175.815720536334));
#14845=CARTESIAN_POINT('Ctrl Pts',(-52.5606356723736,-2.73100846880393,
175.434725535823));
#14846=CARTESIAN_POINT('Ctrl Pts',(-53.1578253291134,-2.60958353788362,
174.986380686329));
#14847=CARTESIAN_POINT('Ctrl Pts',(-53.575919582614,-2.57427864177586,174.934476257966));
#14848=CARTESIAN_POINT('Ctrl Pts',(-54.2645385526377,-2.47204238084449,
175.223470220004));
#14849=CARTESIAN_POINT('Ctrl Pts',(-54.5189943505689,-2.4021627120238,175.561903562137));
#14850=CARTESIAN_POINT('Ctrl Pts',(-54.5814297773468,-2.25612793931688,
176.045419377677));
#14851=CARTESIAN_POINT('Ctrl Pts',(-54.5735173041519,-2.21013144506474,
176.178993521001));
#14852=CARTESIAN_POINT('Ctrl Pts',(-54.5239654997844,-2.13806319233694,
176.36226950621));
#14853=CARTESIAN_POINT('Ctrl Pts',(-54.5010361022764,-2.1121733501921,176.42270110964));
#14854=CARTESIAN_POINT('Ctrl Pts',(-54.4586925003588,-2.07172971741335,
176.508171829538));
#14855=CARTESIAN_POINT('Ctrl Pts',(-54.4432559654462,-2.05799768545568,
176.53580222906));
#14856=CARTESIAN_POINT('Ctrl Pts',(-54.410122331684,-2.03029642349882,176.588723178982));
#14857=CARTESIAN_POINT('Ctrl Pts',(-54.3884821434676,-2.0139079395113,176.618668306411));
#14858=CARTESIAN_POINT('Ctrl Pts',(-54.3738267566562,-2.00237092626598,
176.637865020199));
#14859=CARTESIAN_POINT('Ctrl Pts',(-49.6057233026533,-28.1882175989763,
177.068114089093));
#14860=CARTESIAN_POINT('Ctrl Pts',(-49.5663192275732,-28.1656109096198,
177.105925367078));
#14861=CARTESIAN_POINT('Ctrl Pts',(-49.5216854287654,-28.1457023853521,
177.148383027181));
#14862=CARTESIAN_POINT('Ctrl Pts',(-49.4301127133764,-28.1014695235449,
177.220446553382));
#14863=CARTESIAN_POINT('Ctrl Pts',(-49.3819809603125,-28.0788363277035,
177.253617740645));
#14864=CARTESIAN_POINT('Ctrl Pts',(-49.2321484222821,-28.0099337266433,
177.343479018307));
#14865=CARTESIAN_POINT('Ctrl Pts',(-49.1254026293825,-27.9629901656525,
177.390284377819));
#14866=CARTESIAN_POINT('Ctrl Pts',(-48.7929164986652,-27.8189908160803,
177.48590296908));
#14867=CARTESIAN_POINT('Ctrl Pts',(-48.55635218661,-27.7202377019268,177.490394220553));
#14868=CARTESIAN_POINT('Ctrl Pts',(-47.8840648999533,-27.4305281812212,
177.324447440169));
#14869=CARTESIAN_POINT('Ctrl Pts',(-47.5006474873523,-27.2497443022818,
176.963331771584));
#14870=CARTESIAN_POINT('Ctrl Pts',(-47.2040861213115,-26.9802047380462,
176.046394548579));
#14871=CARTESIAN_POINT('Ctrl Pts',(-47.2954018922066,-26.8917044501032,
175.506598760119));
#14872=CARTESIAN_POINT('Ctrl Pts',(-47.9062028356891,-26.7943163650827,
174.710326627486));
#14873=CARTESIAN_POINT('Ctrl Pts',(-48.4108882632775,-26.7850298620733,
174.47568647468));
#14874=CARTESIAN_POINT('Ctrl Pts',(-49.4081207961382,-26.7654318876047,
174.522051214009));
#14875=CARTESIAN_POINT('Ctrl Pts',(-49.8895805322777,-26.7512165827191,
174.803706734764));
#14876=CARTESIAN_POINT('Ctrl Pts',(-50.419859907048,-26.6406327974915,175.641132157405));
#14877=CARTESIAN_POINT('Ctrl Pts',(-50.4638072135826,-26.5414518590087,
176.190943138814));
#14878=CARTESIAN_POINT('Ctrl Pts',(-50.0902675056585,-26.258306693899,177.06820282525));
#14879=CARTESIAN_POINT('Ctrl Pts',(-49.6753169680471,-26.0710530131776,
177.393289133135));
#14880=CARTESIAN_POINT('Ctrl Pts',(-48.760110273011,-25.6803067135432,177.526354227003));
#14881=CARTESIAN_POINT('Ctrl Pts',(-48.2752065557733,-25.4795815288234,
177.333261554155));
#14882=CARTESIAN_POINT('Ctrl Pts',(-47.6834949732814,-25.1537104488559,
176.598820399841));
#14883=CARTESIAN_POINT('Ctrl Pts',(-47.581935800625,-25.0274199406948,176.066471856633));
#14884=CARTESIAN_POINT('Ctrl Pts',(-47.8743577335121,-24.8702793490883,
175.122570330099));
#14885=CARTESIAN_POINT('Ctrl Pts',(-48.2639300332364,-24.8386062285325,
174.72605490093));
#14886=CARTESIAN_POINT('Ctrl Pts',(-49.2134664973944,-24.8097944361078,
174.418869413643));
#14887=CARTESIAN_POINT('Ctrl Pts',(-49.7639560285487,-24.8089577046691,
174.513086690221));
#14888=CARTESIAN_POINT('Ctrl Pts',(-50.5601436025432,-24.7482854574026,
175.121296078095));
#14889=CARTESIAN_POINT('Ctrl Pts',(-50.7937850628585,-24.6861522884041,
175.625415363842));
#14890=CARTESIAN_POINT('Ctrl Pts',(-50.7513118113109,-24.4660502953853,
176.598470930813));
#14891=CARTESIAN_POINT('Ctrl Pts',(-50.4787452748198,-24.3068424850894,
177.056448064075));
#14892=CARTESIAN_POINT('Ctrl Pts',(-49.6755858463959,-23.9384579984121,
177.525629368769));
#14893=CARTESIAN_POINT('Ctrl Pts',(-49.1583261106009,-23.7318611386462,
177.529378707235));
#14894=CARTESIAN_POINT('Ctrl Pts',(-48.3492917504345,-23.3639427741862,
177.074636497803));
#14895=CARTESIAN_POINT('Ctrl Pts',(-48.0678997211374,-23.2027238239874,
176.620161976926));
#14896=CARTESIAN_POINT('Ctrl Pts',(-48.0133698591323,-22.9779683240005,
175.643265853549));
#14897=CARTESIAN_POINT('Ctrl Pts',(-48.2419634078688,-22.9148026311583,
175.13669620061));
#14898=CARTESIAN_POINT('Ctrl Pts',(-49.0648716087653,-22.8512007031896,
174.491772947554));
#14899=CARTESIAN_POINT('Ctrl Pts',(-49.6839608902416,-22.8528771386521,
174.405900021421));
#14900=CARTESIAN_POINT('Ctrl Pts',(-50.6991943315865,-22.8143164724711,
174.826217042058));
#14901=CARTESIAN_POINT('Ctrl Pts',(-51.0745700439279,-22.7701586995258,
175.322569579276));
#14902=CARTESIAN_POINT('Ctrl Pts',(-51.2073695092728,-22.5604456438022,
176.396956445951));
#14903=CARTESIAN_POINT('Ctrl Pts',(-50.9625278765238,-22.3963905325425,
176.94851178212));
#14904=CARTESIAN_POINT('Ctrl Pts',(-50.1139689940341,-21.9977514714476,
177.529315681618));
#14905=CARTESIAN_POINT('Ctrl Pts',(-49.5293219694751,-21.7666067892758,
177.544699935169));
#14906=CARTESIAN_POINT('Ctrl Pts',(-48.6567664449969,-21.3653910132907,
177.013098304479));
#14907=CARTESIAN_POINT('Ctrl Pts',(-48.383128531039,-21.1949054338945,176.477577858981));
#14908=CARTESIAN_POINT('Ctrl Pts',(-48.4582777380059,-20.975048733324,175.402873064259));
#14909=CARTESIAN_POINT('Ctrl Pts',(-48.8055781932514,-20.9254744005303,
174.886960050279));
#14910=CARTESIAN_POINT('Ctrl Pts',(-49.7998797569528,-20.8818943796597,
174.412232108109));
#14911=CARTESIAN_POINT('Ctrl Pts',(-50.4230224397188,-20.885216808613,174.464849386198));
#14912=CARTESIAN_POINT('Ctrl Pts',(-51.3220781362712,-20.8236066704411,
175.100442044691));
#14913=CARTESIAN_POINT('Ctrl Pts',(-51.5785314568021,-20.7546592125729,
175.670463366294));
#14914=CARTESIAN_POINT('Ctrl Pts',(-51.4682882413066,-20.5004564781585,
176.732562819156));
#14915=CARTESIAN_POINT('Ctrl Pts',(-51.1076577914431,-20.313201754554,177.207532153307));
#14916=CARTESIAN_POINT('Ctrl Pts',(-50.156411198824,-19.8953744930702,177.56803029022));
#14917=CARTESIAN_POINT('Ctrl Pts',(-49.5878400685962,-19.6691878319784,
177.446385146947));
#14918=CARTESIAN_POINT('Ctrl Pts',(-48.852079415717,-19.2920053425884,176.716949064536));
#14919=CARTESIAN_POINT('Ctrl Pts',(-48.7034574890464,-19.1464856081966,
176.127114392609));
#14920=CARTESIAN_POINT('Ctrl Pts',(-49.017896392823,-18.9721498737463,175.084671234462));
#14921=CARTESIAN_POINT('Ctrl Pts',(-49.4761175027563,-18.9421345006494,
174.655217811997));
#14922=CARTESIAN_POINT('Ctrl Pts',(-50.5469446991098,-18.915664221674,174.415005106013));
#14923=CARTESIAN_POINT('Ctrl Pts',(-51.1421889783774,-18.9127734302845,
174.605352538579));
#14924=CARTESIAN_POINT('Ctrl Pts',(-51.8771202801842,-18.8200557591642,
175.418505113175));
#14925=CARTESIAN_POINT('Ctrl Pts',(-52.0018165496213,-18.7275436462981,
176.022835099282));
#14926=CARTESIAN_POINT('Ctrl Pts',(-51.6614363875286,-18.4266465795959,
177.027259608014));
#14927=CARTESIAN_POINT('Ctrl Pts',(-51.2055166082591,-18.2218754080822,
177.403206831321));
#14928=CARTESIAN_POINT('Ctrl Pts',(-50.1969770591628,-17.7923688711786,
177.524973109627));
#14929=CARTESIAN_POINT('Ctrl Pts',(-49.6679526067506,-17.5720619524455,
177.267256975221));
#14930=CARTESIAN_POINT('Ctrl Pts',(-49.1179984398299,-17.2329564925234,
176.379271882249));
#14931=CARTESIAN_POINT('Ctrl Pts',(-49.1058293111544,-17.1129691055462,
175.766207634738));
#14932=CARTESIAN_POINT('Ctrl Pts',(-49.6421979468107,-16.981953011196,174.814805282058));
#14933=CARTESIAN_POINT('Ctrl Pts',(-50.1794692968359,-16.96896833752,174.497498655776));
#14934=CARTESIAN_POINT('Ctrl Pts',(-51.2815033366288,-16.9462509137644,
174.497183387712));
#14935=CARTESIAN_POINT('Ctrl Pts',(-51.8206810039433,-16.9333636766774,
174.813868002799));
#14936=CARTESIAN_POINT('Ctrl Pts',(-52.3579329121243,-16.8019633847227,
175.767995550527));
#14937=CARTESIAN_POINT('Ctrl Pts',(-52.3444015552563,-16.6811074119364,
176.384253300385));
#14938=CARTESIAN_POINT('Ctrl Pts',(-51.7908025496479,-16.3412377353734,
177.270036214878));
#14939=CARTESIAN_POINT('Ctrl Pts',(-51.2640575414935,-16.1220052064028,
177.524939199898));
#14940=CARTESIAN_POINT('Ctrl Pts',(-50.2584821099884,-15.6936926334193,
177.402964762685));
#14941=CARTESIAN_POINT('Ctrl Pts',(-49.8024659570259,-15.4891340123335,
177.028965203342));
#14942=CARTESIAN_POINT('Ctrl Pts',(-49.4615190985809,-15.1881425443655,
176.024838210267));
#14943=CARTESIAN_POINT('Ctrl Pts',(-49.584917871472,-15.0951235636284,175.418993178211));
#14944=CARTESIAN_POINT('Ctrl Pts',(-50.3224323861862,-15.0022736039987,
174.603877612758));
#14945=CARTESIAN_POINT('Ctrl Pts',(-50.9209588419739,-14.9994851008446,
174.413907495741));
#14946=CARTESIAN_POINT('Ctrl Pts',(-51.9913299824675,-14.9728180278691,
174.658436700836));
#14947=CARTESIAN_POINT('Ctrl Pts',(-52.4458562262816,-14.942768055369,175.086526075902));
#14948=CARTESIAN_POINT('Ctrl Pts',(-52.7589234637054,-14.768747576336,176.126312497655));
#14949=CARTESIAN_POINT('Ctrl Pts',(-52.6119738826496,-14.6237809758753,
176.715478760326));
#14950=CARTESIAN_POINT('Ctrl Pts',(-51.8767097042875,-14.2467264136774,
177.445252299972));
#14951=CARTESIAN_POINT('Ctrl Pts',(-51.3074205647036,-14.0201741438431,
177.568755188896));
#14952=CARTESIAN_POINT('Ctrl Pts',(-50.3534291722187,-13.6011459302421,
177.20657523661));
#14953=CARTESIAN_POINT('Ctrl Pts',(-49.9921349812078,-13.4131957453291,
176.728222347554));
#14954=CARTESIAN_POINT('Ctrl Pts',(-49.8860852889645,-13.159806046502,175.66552302478));
#14955=CARTESIAN_POINT('Ctrl Pts',(-50.1425376823364,-13.0914495220188,
175.099033652958));
#14956=CARTESIAN_POINT('Ctrl Pts',(-51.0393482876635,-13.0300320803285,
174.465742160163));
#14957=CARTESIAN_POINT('Ctrl Pts',(-51.661049564308,-13.0333384108268,174.411629490546));
#14958=CARTESIAN_POINT('Ctrl Pts',(-52.6556849728402,-12.9898139344045,
174.885756683857));
#14959=CARTESIAN_POINT('Ctrl Pts',(-53.0050117718212,-12.9403514819039,
175.401975295897));
#14960=CARTESIAN_POINT('Ctrl Pts',(-53.0797917942593,-12.7198628954119,
176.47950485369));
#14961=CARTESIAN_POINT('Ctrl Pts',(-52.8035180796908,-12.5482535501767,
177.017249165378));
#14962=CARTESIAN_POINT('Ctrl Pts',(-51.928756778869,-12.1465816152287,177.545168184464));
#14963=CARTESIAN_POINT('Ctrl Pts',(-51.3476399628683,-11.9168238447545,
177.52855345072));
#14964=CARTESIAN_POINT('Ctrl Pts',(-50.5013329357435,-11.5191203268418,
176.948730973903));
#14965=CARTESIAN_POINT('Ctrl Pts',(-50.2557375091139,-11.3551615877155,
176.398843509589));
#14966=CARTESIAN_POINT('Ctrl Pts',(-50.3877927376681,-11.145398461788,175.324825412843));
#14967=CARTESIAN_POINT('Ctrl Pts',(-50.762684868614,-11.1008426423184,174.826271833705));
#14968=CARTESIAN_POINT('Ctrl Pts',(-51.7811268292925,-11.0622619854364,
174.405264562934));
#14969=CARTESIAN_POINT('Ctrl Pts',(-52.4028793467296,-11.063958202758,174.492793292778));
#14970=CARTESIAN_POINT('Ctrl Pts',(-53.2632154661256,-10.9967409315864,
175.172494096186));
#14971=CARTESIAN_POINT('Ctrl Pts',(-53.4886849878534,-10.9225114509841,
175.750866168407));
#14972=CARTESIAN_POINT('Ctrl Pts',(-53.3251423960266,-10.6565821386363,
176.805379202472));
#14973=CARTESIAN_POINT('Ctrl Pts',(-52.9407422532226,-10.465785944074,177.259010843821));
#14974=CARTESIAN_POINT('Ctrl Pts',(-51.9697953271392,-10.0433159226031,
177.565260787091));
#14975=CARTESIAN_POINT('Ctrl Pts',(-51.4073968434514,-9.81808614025534,
177.411394538556));
#14976=CARTESIAN_POINT('Ctrl Pts',(-50.7116066211125,-9.44884954788431,
176.639139203566));
#14977=CARTESIAN_POINT('Ctrl Pts',(-50.5960828064805,-9.30833579234248,
176.038056438509));
#14978=CARTESIAN_POINT('Ctrl Pts',(-50.9640903737478,-9.14636922546571,
175.0167568496));
#14979=CARTESIAN_POINT('Ctrl Pts',(-51.4414488535671,-9.12058052193367,
174.612974652851));
#14980=CARTESIAN_POINT('Ctrl Pts',(-52.5249204417031,-9.09513784416194,
174.426509843431));
#14981=CARTESIAN_POINT('Ctrl Pts',(-53.1088418277628,-9.09114996369398,
174.646804488947));
#14982=CARTESIAN_POINT('Ctrl Pts',(-53.801661971168,-8.98942785386125,175.498626413927));
#14983=CARTESIAN_POINT('Ctrl Pts',(-53.8945655335682,-8.89052591977855,
176.108945227942));
#14984=CARTESIAN_POINT('Ctrl Pts',(-53.5007325042087,-8.57967938234873,
177.090495387502));
#14985=CARTESIAN_POINT('Ctrl Pts',(-53.0228734977247,-8.36926263084827,
177.439659990072));
#14986=CARTESIAN_POINT('Ctrl Pts',(-52.0134388460396,-7.941561484533,177.502665384752));
#14987=CARTESIAN_POINT('Ctrl Pts',(-51.5009539686643,-7.72503451842822,
177.217498325365));
#14988=CARTESIAN_POINT('Ctrl Pts',(-50.9958226444158,-7.39311721565184,
176.298072843289));
#14989=CARTESIAN_POINT('Ctrl Pts',(-51.0149583411939,-7.28021855779389,
175.684524900703));
#14990=CARTESIAN_POINT('Ctrl Pts',(-51.602189663565,-7.15816051285745,174.759352960774));
#14991=CARTESIAN_POINT('Ctrl Pts',(-52.1561751142271,-7.14821693453925,
174.470064567704));
#14992=CARTESIAN_POINT('Ctrl Pts',(-53.257284967077,-7.12553378294388,174.528734890764));
#14993=CARTESIAN_POINT('Ctrl Pts',(-53.7798318899166,-7.10813319884164,
174.876062446534));
#14994=CARTESIAN_POINT('Ctrl Pts',(-54.263309402104,-6.96831483361839,175.852098283111));
#14995=CARTESIAN_POINT('Ctrl Pts',(-54.2182177005742,-6.84182185515181,
176.463118413));
#14996=CARTESIAN_POINT('Ctrl Pts',(-53.620326169719,-6.49215310837908,177.317242942806));
#14997=CARTESIAN_POINT('Ctrl Pts',(-53.0815432796407,-6.27162057701451,
177.542753252723));
#14998=CARTESIAN_POINT('Ctrl Pts',(-52.0813405764902,-5.84340716815714,
177.363069610828));
#14999=CARTESIAN_POINT('Ctrl Pts',(-51.6451899827477,-5.64252013198273,
176.962963727015));
#15000=CARTESIAN_POINT('Ctrl Pts',(-51.3585173428123,-5.35236886702559,
175.939011043839));
#15001=CARTESIAN_POINT('Ctrl Pts',(-51.5164782073777,-5.2645103327986,175.337256223397));
#15002=CARTESIAN_POINT('Ctrl Pts',(-52.2924300679745,-5.18119763163266,
174.565366155634));
#15003=CARTESIAN_POINT('Ctrl Pts',(-52.8973452213176,-5.1801045826173,174.406680096152));
#15004=CARTESIAN_POINT('Ctrl Pts',(-53.956162505713,-5.14973256956073,174.705214074754));
#15005=CARTESIAN_POINT('Ctrl Pts',(-54.3874707400874,-5.11629663400306,
175.155234787811));
#15006=CARTESIAN_POINT('Ctrl Pts',(-54.6460006492434,-4.93091655090319,
176.210608238885));
#15007=CARTESIAN_POINT('Ctrl Pts',(-54.4681690759566,-4.77980797892323,
176.790635503925));
#15008=CARTESIAN_POINT('Ctrl Pts',(-53.6946945331643,-4.3956772156615,177.47627897342));
#15009=CARTESIAN_POINT('Ctrl Pts',(-53.1174419759953,-4.16620647621949,
177.565792133827));
#15010=CARTESIAN_POINT('Ctrl Pts',(-52.1878574222778,-3.75385530866336,
177.150829002666));
#15011=CARTESIAN_POINT('Ctrl Pts',(-51.8529856411974,-3.5715083216093,176.654958973924));
#15012=CARTESIAN_POINT('Ctrl Pts',(-51.8010050251376,-3.32706416715232,
175.583828138226));
#15013=CARTESIAN_POINT('Ctrl Pts',(-52.0854219579878,-3.26527816982496,
175.031488604324));
#15014=CARTESIAN_POINT('Ctrl Pts',(-53.0170398348192,-3.20959915076688,
174.444132662069));
#15015=CARTESIAN_POINT('Ctrl Pts',(-53.6416591927321,-3.21325709639781,
174.423035709656));
#15016=CARTESIAN_POINT('Ctrl Pts',(-54.6090153740635,-3.16498595686182,
174.948967905512));
#15017=CARTESIAN_POINT('Ctrl Pts',(-54.9308286711417,-3.10893139642228,
175.48555871107));
#15018=CARTESIAN_POINT('Ctrl Pts',(-54.9426665516143,-2.95192631073098,
176.218540695264));
#15019=CARTESIAN_POINT('Ctrl Pts',(-54.9070365263685,-2.90171640292054,
176.413787336324));
#15020=CARTESIAN_POINT('Ctrl Pts',(-54.8013987998623,-2.81782847468563,
176.681821034794));
#15021=CARTESIAN_POINT('Ctrl Pts',(-54.7570848510793,-2.78787367953458,
176.767627228561));
#15022=CARTESIAN_POINT('Ctrl Pts',(-54.6793253219128,-2.74078668455889,
176.887592985838));
#15023=CARTESIAN_POINT('Ctrl Pts',(-54.651529701944,-2.72473899696222,176.926133356148));
#15024=CARTESIAN_POINT('Ctrl Pts',(-54.5925997439423,-2.69209575899625,
176.999824075839));
#15025=CARTESIAN_POINT('Ctrl Pts',(-54.5641015373143,-2.67654794454284,
177.031971691023));
#15026=CARTESIAN_POINT('Ctrl Pts',(-54.5288628436534,-2.65870383148503,
177.068203177065));
#15027=CARTESIAN_POINT('Ctrl Pts',(-49.7605161567837,-28.8447111186158,
177.498294784826));
#15028=CARTESIAN_POINT('Ctrl Pts',(-49.703499066658,-28.8235655424673,177.540214005203));
#15029=CARTESIAN_POINT('Ctrl Pts',(-49.6410455761305,-28.7951782353542,
177.600452889938));
#15030=CARTESIAN_POINT('Ctrl Pts',(-49.5125749804916,-28.7439261033728,
177.690427833332));
#15031=CARTESIAN_POINT('Ctrl Pts',(-49.4455382815264,-28.7177519743038,
177.731297783696));
#15032=CARTESIAN_POINT('Ctrl Pts',(-49.2376911387288,-28.6378112833129,
177.840935439774));
#15033=CARTESIAN_POINT('Ctrl Pts',(-49.0899159828253,-28.5824382846613,
177.897035937477));
#15034=CARTESIAN_POINT('Ctrl Pts',(-48.6337896696199,-28.4146446752159,
178.002589339604));
#15035=CARTESIAN_POINT('Ctrl Pts',(-48.3132270959126,-28.2997217083806,
177.992428880102));
#15036=CARTESIAN_POINT('Ctrl Pts',(-47.4162097247782,-27.9673749676665,
177.725331904959));
#15037=CARTESIAN_POINT('Ctrl Pts',(-46.9189492851719,-27.7652251395226,
177.218083285283));
#15038=CARTESIAN_POINT('Ctrl Pts',(-46.5632291525645,-27.4820421855238,
175.966063107167));
#15039=CARTESIAN_POINT('Ctrl Pts',(-46.7140098167225,-27.4055520605101,
175.249184591433));
#15040=CARTESIAN_POINT('Ctrl Pts',(-47.566085933826,-27.3558389712614,174.223160308952));
#15041=CARTESIAN_POINT('Ctrl Pts',(-48.2470586621674,-27.3810915115113,
173.939995635501));
#15042=CARTESIAN_POINT('Ctrl Pts',(-49.5700361455588,-27.4220834505067,
174.062399212278));
#15043=CARTESIAN_POINT('Ctrl Pts',(-50.1884067287968,-27.434811958294,174.470377906696));
#15044=CARTESIAN_POINT('Ctrl Pts',(-50.8303308863031,-27.3468909642006,
175.620618298056));
#15045=CARTESIAN_POINT('Ctrl Pts',(-50.8493116919004,-27.2434061722865,
176.356125167609));
#15046=CARTESIAN_POINT('Ctrl Pts',(-50.2816569479994,-26.9206929510016,
177.507808537998));
#15047=CARTESIAN_POINT('Ctrl Pts',(-49.6987348616025,-26.7015350212598,
177.912925525668));
#15048=CARTESIAN_POINT('Ctrl Pts',(-48.454710251186,-26.2485207329848,178.028292067179));
#15049=CARTESIAN_POINT('Ctrl Pts',(-47.8121824616331,-26.017945810327,177.739239128205));
#15050=CARTESIAN_POINT('Ctrl Pts',(-47.0491566977328,-25.6568136786021,
176.713556301102));
#15051=CARTESIAN_POINT('Ctrl Pts',(-46.9415518318806,-25.5298970910749,
175.993584668982));
#15052=CARTESIAN_POINT('Ctrl Pts',(-47.3778834474909,-25.4016448622981,
174.749674324357));
#15053=CARTESIAN_POINT('Ctrl Pts',(-47.9149438708112,-25.3989201973124,
174.243242130538));
#15054=CARTESIAN_POINT('Ctrl Pts',(-49.195098595239,-25.4317364372956,173.888113334518));
#15055=CARTESIAN_POINT('Ctrl Pts',(-49.918185567551,-25.4646653275392,174.050133776974));
#15056=CARTESIAN_POINT('Ctrl Pts',(-50.9295131393841,-25.4466210128473,
174.911633886668));
#15057=CARTESIAN_POINT('Ctrl Pts',(-51.2044913533823,-25.3930064438348,
175.597822621196));
#15058=CARTESIAN_POINT('Ctrl Pts',(-51.0754639563939,-25.1539869007477,
176.899089439364));
#15059=CARTESIAN_POINT('Ctrl Pts',(-50.6742118208058,-24.9705041413757,
177.491449801663));
#15060=CARTESIAN_POINT('Ctrl Pts',(-49.5587075034334,-24.5430242840169,
178.062955652865));
#15061=CARTESIAN_POINT('Ctrl Pts',(-48.8611723259578,-24.3021716495128,
178.034645386427));
#15062=CARTESIAN_POINT('Ctrl Pts',(-47.7896195282427,-23.8814983836082,
177.370866230542));
#15063=CARTESIAN_POINT('Ctrl Pts',(-47.4363508410467,-23.7069028048269,
176.742728542957));
#15064=CARTESIAN_POINT('Ctrl Pts',(-47.4114253180649,-23.4889969329168,
175.432113003805));
#15065=CARTESIAN_POINT('Ctrl Pts',(-47.740070725129,-23.4456714422117,174.768834597493));
#15066=CARTESIAN_POINT('Ctrl Pts',(-48.8702204177861,-23.4389819923271,
173.952056567371));
#15067=CARTESIAN_POINT('Ctrl Pts',(-49.6947930376395,-23.4814638927378,
173.877925688461));
#15068=CARTESIAN_POINT('Ctrl Pts',(-51.0112605873021,-23.5013279450334,
174.502758507842));
#15069=CARTESIAN_POINT('Ctrl Pts',(-51.4766740890821,-23.4736078700863,
175.190881305064));
#15070=CARTESIAN_POINT('Ctrl Pts',(-51.5715098854918,-23.2578265151817,
176.631332013987));
#15071=CARTESIAN_POINT('Ctrl Pts',(-51.2026984232359,-23.0689810535093,
177.353708555585));
#15072=CARTESIAN_POINT('Ctrl Pts',(-50.0169981786826,-22.6055963153184,
178.072791197941));
#15073=CARTESIAN_POINT('Ctrl Pts',(-49.2289032454779,-22.3364394885883,
178.054791801573));
#15074=CARTESIAN_POINT('Ctrl Pts',(-48.0752306219957,-21.8785657833076,
177.283552800795));
#15075=CARTESIAN_POINT('Ctrl Pts',(-47.7373875210752,-21.6968802590999,
176.548566639058));
#15076=CARTESIAN_POINT('Ctrl Pts',(-47.8901343487967,-21.492320838371,175.113663385513));
#15077=CARTESIAN_POINT('Ctrl Pts',(-48.3804128007365,-21.4693940830233,
174.442825661914));
#15078=CARTESIAN_POINT('Ctrl Pts',(-49.7230759786915,-21.4942443138953,
173.870938911605));
#15079=CARTESIAN_POINT('Ctrl Pts',(-50.5477501626655,-21.53554466513,173.979304242753));
#15080=CARTESIAN_POINT('Ctrl Pts',(-51.6956775721548,-21.5221965965903,
174.884495307656));
#15081=CARTESIAN_POINT('Ctrl Pts',(-51.995185395164,-21.4627711751308,175.65946330393));
#15082=CARTESIAN_POINT('Ctrl Pts',(-51.7684808698132,-21.1836626405178,
177.075777271268));
#15083=CARTESIAN_POINT('Ctrl Pts',(-51.248410167092,-20.9668436684778,177.683928269078));
#15084=CARTESIAN_POINT('Ctrl Pts',(-49.9393032270381,-20.4803392816045,
178.101596183419));
#15085=CARTESIAN_POINT('Ctrl Pts',(-49.1773119956809,-20.2159303489599,
177.900701030808));
#15086=CARTESIAN_POINT('Ctrl Pts',(-48.2258296454727,-19.7984008812386,
176.875814996871));
#15087=CARTESIAN_POINT('Ctrl Pts',(-48.0552229745052,-19.6477554978605,
176.074637438704));
#15088=CARTESIAN_POINT('Ctrl Pts',(-48.5258258225559,-19.5038059294262,
174.698094313544));
#15089=CARTESIAN_POINT('Ctrl Pts',(-49.1555523948045,-19.5080820109078,
174.15313676254));
#15090=CARTESIAN_POINT('Ctrl Pts',(-50.5933891726929,-19.5499376382275,
173.895161972129));
#15091=CARTESIAN_POINT('Ctrl Pts',(-51.368058411907,-19.5828296420673,174.188177381599));
#15092=CARTESIAN_POINT('Ctrl Pts',(-52.285250485287,-19.5255903568737,175.320127767442));
#15093=CARTESIAN_POINT('Ctrl Pts',(-52.4079017329002,-19.4317611692977,
176.136959370172));
#15094=CARTESIAN_POINT('Ctrl Pts',(-51.8753008807154,-19.0950488584311,
177.453114298066));
#15095=CARTESIAN_POINT('Ctrl Pts',(-51.2342686483785,-18.8536936439763,
177.926872571079));
#15096=CARTESIAN_POINT('Ctrl Pts',(-49.8632157867063,-18.3545541183897,
178.021760725256));
#15097=CARTESIAN_POINT('Ctrl Pts',(-49.1660096364335,-18.1030331017558,
177.643137201611));
#15098=CARTESIAN_POINT('Ctrl Pts',(-48.4670297183309,-17.7327410070788,
176.413682699456));
#15099=CARTESIAN_POINT('Ctrl Pts',(-48.483334940274,-17.6194284897493,175.592916154309));
#15100=CARTESIAN_POINT('Ctrl Pts',(-49.2450668681383,-17.5322013902257,
174.352697167155));
#15101=CARTESIAN_POINT('Ctrl Pts',(-49.9777722871607,-17.5559821453049,
173.960304681794));
#15102=CARTESIAN_POINT('Ctrl Pts',(-51.4344516507071,-17.6029063882428,
174.028937019837));
#15103=CARTESIAN_POINT('Ctrl Pts',(-52.1305828574604,-17.6193975644539,
174.485906049309));
#15104=CARTESIAN_POINT('Ctrl Pts',(-52.774838706301,-17.5089074046146,175.793694056009));
#15105=CARTESIAN_POINT('Ctrl Pts',(-52.7115258732458,-17.3796686755426,
176.613178448276));
#15106=CARTESIAN_POINT('Ctrl Pts',(-51.9002446822929,-16.9876585431162,
177.764926590858));
#15107=CARTESIAN_POINT('Ctrl Pts',(-51.1728057089079,-16.7309097600974,
178.068009087089));
#15108=CARTESIAN_POINT('Ctrl Pts',(-49.8211348979667,-16.2361848829689,
177.837068581403));
#15109=CARTESIAN_POINT('Ctrl Pts',(-49.2256314668982,-16.0038069200319,
177.305047152795));
#15110=CARTESIAN_POINT('Ctrl Pts',(-48.8186328386387,-15.691330495564,175.939125806104));
#15111=CARTESIAN_POINT('Ctrl Pts',(-49.013546517339,-15.6112127223192,175.133605172695));
#15112=CARTESIAN_POINT('Ctrl Pts',(-50.0357499087345,-15.5735396207079,
174.088389632472));
#15113=CARTESIAN_POINT('Ctrl Pts',(-50.8379174497137,-15.6112366284576,
173.871670522767));
#15114=CARTESIAN_POINT('Ctrl Pts',(-52.2457834487726,-15.6472027358935,
174.26447248136));
#15115=CARTESIAN_POINT('Ctrl Pts',(-52.8170337247495,-15.6408479370702,
174.8653310014));
#15116=CARTESIAN_POINT('Ctrl Pts',(-53.1560440051794,-15.4721566908598,
176.273031298879));
#15117=CARTESIAN_POINT('Ctrl Pts',(-52.9154253174859,-15.3082073561117,
177.052126824288));
#15118=CARTESIAN_POINT('Ctrl Pts',(-51.8728096300678,-14.8731360568539,
177.975770830197));
#15119=CARTESIAN_POINT('Ctrl Pts',(-51.0951645133176,-14.6055143185424,
178.104087436367));
#15120=CARTESIAN_POINT('Ctrl Pts',(-49.8271933090145,-14.1262171391814,
177.555333624295));
#15121=CARTESIAN_POINT('Ctrl Pts',(-49.3671436709228,-13.9204374671742,
176.893150416479));
#15122=CARTESIAN_POINT('Ctrl Pts',(-49.274728926638,-13.6672296225191,175.457007277905));
#15123=CARTESIAN_POINT('Ctrl Pts',(-49.6465886024413,-13.6223148063404,
174.716642572685));
#15124=CARTESIAN_POINT('Ctrl Pts',(-50.8704338551746,-13.6242867085274,
173.925061362222));
#15125=CARTESIAN_POINT('Ctrl Pts',(-51.7000786840932,-13.666773744136,173.890948850678));
#15126=CARTESIAN_POINT('Ctrl Pts',(-52.983493848767,-13.6801901085456,174.58610021153));
#15127=CARTESIAN_POINT('Ctrl Pts',(-53.4130967944053,-13.6453172862449,
175.298527478907));
#15128=CARTESIAN_POINT('Ctrl Pts',(-53.4312271360186,-13.4141834163833,
176.741466379681));
#15129=CARTESIAN_POINT('Ctrl Pts',(-53.0223631213944,-13.2182197961852,
177.439586265974));
#15130=CARTESIAN_POINT('Ctrl Pts',(-51.8015717929752,-12.7473718779738,
178.090703687822));
#15131=CARTESIAN_POINT('Ctrl Pts',(-51.0193050555008,-12.4800112867217,
178.027617006182));
#15132=CARTESIAN_POINT('Ctrl Pts',(-49.9091230827754,-12.0317475039094,
177.194798446979));
#15133=CARTESIAN_POINT('Ctrl Pts',(-49.6065982226317,-11.8558917537395,
176.440442987632));
#15134=CARTESIAN_POINT('Ctrl Pts',(-49.8356019855053,-11.6660764580159,
175.012059004046));
#15135=CARTESIAN_POINT('Ctrl Pts',(-50.3610430198266,-11.6496605652263,
174.366149315963));
#15136=CARTESIAN_POINT('Ctrl Pts',(-51.7343806490719,-11.6797988495863,
173.866104995302));
#15137=CARTESIAN_POINT('Ctrl Pts',(-52.550540790582,-11.7201981252995,174.02088411371));
#15138=CARTESIAN_POINT('Ctrl Pts',(-53.6500640270725,-11.6966559909963,
174.984749041133));
#15139=CARTESIAN_POINT('Ctrl Pts',(-53.9056865612328,-11.6294298688172,
175.770695352483));
#15140=CARTESIAN_POINT('Ctrl Pts',(-53.6065172861421,-11.3376692947806,
177.167270913611));
#15141=CARTESIAN_POINT('Ctrl Pts',(-53.0559160748103,-11.1139055956972,
177.749439639131));
#15142=CARTESIAN_POINT('Ctrl Pts',(-51.7252371686403,-10.6233177496803,
178.092170345976));
#15143=CARTESIAN_POINT('Ctrl Pts',(-50.9736524019596,-10.3607126008384,
177.849203208466));
#15144=CARTESIAN_POINT('Ctrl Pts',(-50.0765013772471,-9.95292884744916,
176.76875224789));
#15145=CARTESIAN_POINT('Ctrl Pts',(-49.9516819265813,-9.81183425780667,
175.958513771998));
#15146=CARTESIAN_POINT('Ctrl Pts',(-50.4932223958658,-9.68088414604229,
174.607725553029));
#15147=CARTESIAN_POINT('Ctrl Pts',(-51.1493491071183,-9.69075789692425,
174.099564788001));
#15148=CARTESIAN_POINT('Ctrl Pts',(-52.5949212007306,-9.73546275490891,
173.917493057606));
#15149=CARTESIAN_POINT('Ctrl Pts',(-53.3569613223681,-9.76490646019358,
174.248860303054));
#15150=CARTESIAN_POINT('Ctrl Pts',(-54.2135986647274,-9.69602761498083,
175.428657754819));
#15151=CARTESIAN_POINT('Ctrl Pts',(-54.293848370144,-9.59379233086061,176.251060243097));
#15152=CARTESIAN_POINT('Ctrl Pts',(-53.6913007216372,-9.24298063305673,
177.535379997424));
#15153=CARTESIAN_POINT('Ctrl Pts',(-53.0251793740895,-8.99747173235245,
177.96924977839));
#15154=CARTESIAN_POINT('Ctrl Pts',(-51.651725273033,-8.49712492600163,177.987723094373));
#15155=CARTESIAN_POINT('Ctrl Pts',(-50.9786512815054,-8.25081939601668,
177.570771429869));
#15156=CARTESIAN_POINT('Ctrl Pts',(-50.3458167934762,-7.89459730610716,
176.305935969218));
#15157=CARTESIAN_POINT('Ctrl Pts',(-50.4021522245058,-7.78795543802409,
175.483191418641));
#15158=CARTESIAN_POINT('Ctrl Pts',(-51.2295886328818,-7.71347110197539,
174.283262770515));
#15159=CARTESIAN_POINT('Ctrl Pts',(-51.9823539758956,-7.74096536711586,
173.929068927273));
#15160=CARTESIAN_POINT('Ctrl Pts',(-53.4363603166253,-7.78662015021704,
174.075813689628));
#15161=CARTESIAN_POINT('Ctrl Pts',(-54.1043459363082,-7.79847651244032,
174.570723179108));
#15162=CARTESIAN_POINT('Ctrl Pts',(-54.6799658608561,-7.67397811007903,
175.90877571489));
#15163=CARTESIAN_POINT('Ctrl Pts',(-54.5722464428634,-7.53659878310187,
176.719948913595));
#15164=CARTESIAN_POINT('Ctrl Pts',(-53.7048106882453,-7.13527023180301,
177.820508243663));
#15165=CARTESIAN_POINT('Ctrl Pts',(-52.9613211614002,-6.87434685741961,
178.086941994317));
#15166=CARTESIAN_POINT('Ctrl Pts',(-51.6221407922901,-6.38201846097514,
177.778890662373));
#15167=CARTESIAN_POINT('Ctrl Pts',(-51.0546870579556,-6.15491662175662,
177.213869145202));
#15168=CARTESIAN_POINT('Ctrl Pts',(-50.7203127232504,-5.85585141799114,
175.823263107997));
#15169=CARTESIAN_POINT('Ctrl Pts',(-50.9602054908589,-5.78500310757108,
175.029480964866));
#15170=CARTESIAN_POINT('Ctrl Pts',(-52.0343424634976,-5.75674450428783,
174.039165918607));
#15171=CARTESIAN_POINT('Ctrl Pts',(-52.8447329543179,-5.79646505952858,
173.866867743832));
#15172=CARTESIAN_POINT('Ctrl Pts',(-54.227093102642,-5.82880399980787,174.331684606762));
#15173=CARTESIAN_POINT('Ctrl Pts',(-54.7703330160768,-5.81603743040407,
174.961265757845));
#15174=CARTESIAN_POINT('Ctrl Pts',(-55.0342584322448,-5.63295034503888,
176.384531023624));
#15175=CARTESIAN_POINT('Ctrl Pts',(-54.7535167216846,-5.46110103683509,
177.149304158576));
#15176=CARTESIAN_POINT('Ctrl Pts',(-53.6617191466184,-5.01587299208642,
178.013397713687));
#15177=CARTESIAN_POINT('Ctrl Pts',(-52.8789563910228,-4.7479816344422,178.094733745787));
#15178=CARTESIAN_POINT('Ctrl Pts',(-51.6416463903481,-4.27383996939189,
177.476508505419));
#15179=CARTESIAN_POINT('Ctrl Pts',(-51.2194660036301,-4.07584859930261,
176.790317421121));
#15180=CARTESIAN_POINT('Ctrl Pts',(-51.2019938075703,-3.83837584139065,
175.351935740118));
#15181=CARTESIAN_POINT('Ctrl Pts',(-51.610208243602,-3.79954787084599,174.628251672824));
#15182=CARTESIAN_POINT('Ctrl Pts',(-52.8762543405249,-3.80961476365013,
173.901884637809));
#15183=CARTESIAN_POINT('Ctrl Pts',(-53.7073988028502,-3.85223555101975,
173.911595161346));
#15184=CARTESIAN_POINT('Ctrl Pts',(-54.9534921954892,-3.85792953287916,
174.67446559102));
#15185=CARTESIAN_POINT('Ctrl Pts',(-55.3426629917145,-3.81570008082077,
175.409213860003));
#15186=CARTESIAN_POINT('Ctrl Pts',(-55.3039033258818,-3.64772468214507,
176.391662012851));
#15187=CARTESIAN_POINT('Ctrl Pts',(-55.240555748585,-3.59330136077634,176.648581151648));
#15188=CARTESIAN_POINT('Ctrl Pts',(-55.0788320999402,-3.49759375703432,
177.001372563377));
#15189=CARTESIAN_POINT('Ctrl Pts',(-55.0131335998823,-3.46357400887706,
177.112553347482));
#15190=CARTESIAN_POINT('Ctrl Pts',(-54.8999581434668,-3.40984365170443,
177.267014142137));
#15191=CARTESIAN_POINT('Ctrl Pts',(-54.8598034384417,-3.39148030846876,
177.316464483235));
#15192=CARTESIAN_POINT('Ctrl Pts',(-54.7750771562006,-3.35389509449369,
177.410924972696));
#15193=CARTESIAN_POINT('Ctrl Pts',(-54.7397209311609,-3.33918794957438,
177.445275075635));
#15194=CARTESIAN_POINT('Ctrl Pts',(-54.6838989306507,-3.31503673670408,
177.498541333932));
#15195=CARTESIAN_POINT('Ctrl Pts',(-50.3479071748434,-28.4569951884828,
177.87862115707));
#15196=CARTESIAN_POINT('Ctrl Pts',(-50.2728575672733,-28.4359962578257,
177.948540001849));
#15197=CARTESIAN_POINT('Ctrl Pts',(-50.1962258409275,-28.4010191615162,
178.021251708215));
#15198=CARTESIAN_POINT('Ctrl Pts',(-50.0327133344336,-28.3431284715803,
178.148112768101));
#15199=CARTESIAN_POINT('Ctrl Pts',(-49.9471957757512,-28.3135226108735,
178.206264690109));
#15200=CARTESIAN_POINT('Ctrl Pts',(-49.6807194301921,-28.2224721023673,
178.364232700982));
#15201=CARTESIAN_POINT('Ctrl Pts',(-49.4886308694229,-28.1579103591893,
178.447943211646));
#15202=CARTESIAN_POINT('Ctrl Pts',(-48.8935956196606,-27.9633647516093,
178.618732735728));
#15203=CARTESIAN_POINT('Ctrl Pts',(-48.4698811368596,-27.8285932845993,
178.628088311833));
#15204=CARTESIAN_POINT('Ctrl Pts',(-47.2704244122812,-27.4388125604887,
178.343093993075));
#15205=CARTESIAN_POINT('Ctrl Pts',(-46.5780488855805,-27.1997688494767,
177.716319207522));
#15206=CARTESIAN_POINT('Ctrl Pts',(-46.0180477417519,-26.8743979377982,
176.099249510754));
#15207=CARTESIAN_POINT('Ctrl Pts',(-46.162624656611,-26.7973830650002,175.153557109113));
#15208=CARTESIAN_POINT('Ctrl Pts',(-47.1953010051746,-26.7839304768722,
173.755742992678));
#15209=CARTESIAN_POINT('Ctrl Pts',(-48.0607153645256,-26.8454387863112,
173.337748493251));
#15210=CARTESIAN_POINT('Ctrl Pts',(-49.7936242958811,-26.9626978867657,
173.412243144396));
#15211=CARTESIAN_POINT('Ctrl Pts',(-50.6218862360795,-27.016572452629,173.905326198308));
#15212=CARTESIAN_POINT('Ctrl Pts',(-51.5258205855669,-26.9805930176338,
175.367177784907));
#15213=CARTESIAN_POINT('Ctrl Pts',(-51.5951438365624,-26.8874613833773,
176.329869003407));
#15214=CARTESIAN_POINT('Ctrl Pts',(-50.9127162462792,-26.5399486517808,
177.882574589842));
#15215=CARTESIAN_POINT('Ctrl Pts',(-50.1707795944383,-26.2907274748939,
178.452449051012));
#15216=CARTESIAN_POINT('Ctrl Pts',(-48.5397246316051,-25.7645038790956,
178.692502082553));
#15217=CARTESIAN_POINT('Ctrl Pts',(-47.67260524551,-25.4913101058597,178.361691922331));
#15218=CARTESIAN_POINT('Ctrl Pts',(-46.5924693917267,-25.0662449204663,
177.069022085109));
#15219=CARTESIAN_POINT('Ctrl Pts',(-46.3991806471167,-24.9234731673228,
176.136653590829));
#15220=CARTESIAN_POINT('Ctrl Pts',(-46.8738389297659,-24.8040321200569,
174.482872284355));
#15221=CARTESIAN_POINT('Ctrl Pts',(-47.5355683392896,-24.8259889159373,
173.783025779917));
#15222=CARTESIAN_POINT('Ctrl Pts',(-49.181078144729,-24.926602323961,173.233424036193));
#15223=CARTESIAN_POINT('Ctrl Pts',(-50.130455303743,-25.0037631556439,173.398086820976));
#15224=CARTESIAN_POINT('Ctrl Pts',(-51.4978889309697,-25.0558147041254,
174.456799989093));
#15225=CARTESIAN_POINT('Ctrl Pts',(-51.8989353348306,-25.0272033256972,
175.336539369917));
#15226=CARTESIAN_POINT('Ctrl Pts',(-51.8018863283238,-24.7915666340119,
177.05629857501));
#15227=CARTESIAN_POINT('Ctrl Pts',(-51.3095767986978,-24.5911935663349,
177.858613821852));
#15228=CARTESIAN_POINT('Ctrl Pts',(-49.8771546536489,-24.10401978861,178.68604557473));
#15229=CARTESIAN_POINT('Ctrl Pts',(-48.9560458718938,-23.8206956072764,
178.700341600297));
#15230=CARTESIAN_POINT('Ctrl Pts',(-47.4944002604164,-23.3221357921539,
177.903717692127));
#15231=CARTESIAN_POINT('Ctrl Pts',(-46.9859140286074,-23.1182050059858,
177.107706307993));
#15232=CARTESIAN_POINT('Ctrl Pts',(-46.8530474021693,-22.8809089149922,
175.398792520737));
#15233=CARTESIAN_POINT('Ctrl Pts',(-47.231059536602,-22.8477944049951,174.508609012772));
#15234=CARTESIAN_POINT('Ctrl Pts',(-48.6493873331158,-22.8937567040743,
173.363150661036));
#15235=CARTESIAN_POINT('Ctrl Pts',(-49.7143921444323,-22.9840542321675,
173.211662996139));
#15236=CARTESIAN_POINT('Ctrl Pts',(-51.4652368913311,-23.0881428692961,
173.941607840096));
#15237=CARTESIAN_POINT('Ctrl Pts',(-52.1136094605607,-23.094525291844,174.813935779811));
#15238=CARTESIAN_POINT('Ctrl Pts',(-52.3204663109761,-22.9019098705719,
176.69350767169));
#15239=CARTESIAN_POINT('Ctrl Pts',(-51.877821743202,-22.6977464609932,177.66752824204));
#15240=CARTESIAN_POINT('Ctrl Pts',(-50.3601753662095,-22.1706433373772,
178.693383453661));
#15241=CARTESIAN_POINT('Ctrl Pts',(-49.3218325614145,-21.8547798388568,
178.72781114664));
#15242=CARTESIAN_POINT('Ctrl Pts',(-47.7441093775104,-21.3120724766084,
177.795709587611));
#15243=CARTESIAN_POINT('Ctrl Pts',(-47.2477760409393,-21.1012761066736,
176.860414332907));
#15244=CARTESIAN_POINT('Ctrl Pts',(-47.3387825873497,-20.8852685243919,
174.97505816188));
#15245=CARTESIAN_POINT('Ctrl Pts',(-47.9314309575524,-20.8809046965219,
174.063915635121));
#15246=CARTESIAN_POINT('Ctrl Pts',(-49.6347357453554,-20.9768646680186,
173.225964829082));
#15247=CARTESIAN_POINT('Ctrl Pts',(-50.7167240875825,-21.0667038014875,
173.313184970442));
#15248=CARTESIAN_POINT('Ctrl Pts',(-52.2657610285106,-21.1310010461024,
174.421840220958));
#15249=CARTESIAN_POINT('Ctrl Pts',(-52.7037384700293,-21.0998274566763,
175.41493210957));
#15250=CARTESIAN_POINT('Ctrl Pts',(-52.4847175837037,-20.8191405044519,
177.292562937125));
#15251=CARTESIAN_POINT('Ctrl Pts',(-51.8386241308113,-20.5794725658491,
178.12361350116));
#15252=CARTESIAN_POINT('Ctrl Pts',(-50.1396663396365,-20.018246073474,178.763454537015));
#15253=CARTESIAN_POINT('Ctrl Pts',(-49.1209540205185,-19.7031542981699,
178.552891694314));
#15254=CARTESIAN_POINT('Ctrl Pts',(-47.794702927651,-19.2149188701855,177.282197399313));
#15255=CARTESIAN_POINT('Ctrl Pts',(-47.5115450575125,-19.0414866308731,
176.244710688925));
#15256=CARTESIAN_POINT('Ctrl Pts',(-48.0225076992042,-18.9056180257745,
174.413639337664));
#15257=CARTESIAN_POINT('Ctrl Pts',(-48.8010517900779,-18.9401402740231,
173.657816206187));
#15258=CARTESIAN_POINT('Ctrl Pts',(-50.6589325202962,-19.0599362479824,
173.225466551806));
#15259=CARTESIAN_POINT('Ctrl Pts',(-51.6828783925415,-19.1423524153639,
173.556811131415));
#15260=CARTESIAN_POINT('Ctrl Pts',(-52.94490571859,-19.1520660317591,174.977944054317));
#15261=CARTESIAN_POINT('Ctrl Pts',(-53.1522316495948,-19.0733891332466,
176.042129261136));
#15262=CARTESIAN_POINT('Ctrl Pts',(-52.5304975170958,-18.7210523123868,
177.802820234119));
#15263=CARTESIAN_POINT('Ctrl Pts',(-51.7144732100097,-18.4448678812944,
178.469420248747));
#15264=CARTESIAN_POINT('Ctrl Pts',(-49.9127782169188,-17.8629843097264,
178.691085462265));
#15265=CARTESIAN_POINT('Ctrl Pts',(-48.9683571282271,-17.5653381811437,
178.247635108413));
#15266=CARTESIAN_POINT('Ctrl Pts',(-47.9579076603942,-17.1319211116872,
176.683402031933));
#15267=CARTESIAN_POINT('Ctrl Pts',(-47.9184077060768,-17.009302655329,175.611974434002));
#15268=CARTESIAN_POINT('Ctrl Pts',(-48.8193204272181,-16.9493687678545,
173.939410793842));
#15269=CARTESIAN_POINT('Ctrl Pts',(-49.7479148095836,-17.0097492793151,
173.377008912436));
#15270=CARTESIAN_POINT('Ctrl Pts',(-51.643208967551,-17.1428193004232,173.368498519432));
#15271=CARTESIAN_POINT('Ctrl Pts',(-52.5796094505093,-17.2045582837911,
173.921665784702));
#15272=CARTESIAN_POINT('Ctrl Pts',(-53.4961681928706,-17.1468816411331,
175.591939966795));
#15273=CARTESIAN_POINT('Ctrl Pts',(-53.4629851797616,-17.024999612415,176.669185388437));
#15274=CARTESIAN_POINT('Ctrl Pts',(-52.4593346223015,-16.5928308404044,
178.238747171052));
#15275=CARTESIAN_POINT('Ctrl Pts',(-51.5224253668316,-16.2971453030902,
178.685547111838));
#15276=CARTESIAN_POINT('Ctrl Pts',(-49.7246467734476,-15.7168449309467,
178.479497386489));
#15277=CARTESIAN_POINT('Ctrl Pts',(-48.9027009029283,-15.4396261238498,
177.823563805929));
#15278=CARTESIAN_POINT('Ctrl Pts',(-48.2654141259822,-15.0843052308904,
176.069175886686));
#15279=CARTESIAN_POINT('Ctrl Pts',(-48.4613159716259,-15.0032908855178,
175.000998038449));
#15280=CARTESIAN_POINT('Ctrl Pts',(-49.7162174501553,-15.01079667333,173.565578406105));
#15281=CARTESIAN_POINT('Ctrl Pts',(-50.7428205977302,-15.0933182852754,
173.226451476554));
#15282=CARTESIAN_POINT('Ctrl Pts',(-52.6035006910652,-15.2135426682566,
173.650512878487));
#15283=CARTESIAN_POINT('Ctrl Pts',(-53.382025542189,-15.2486168447941,174.397702687793));
#15284=CARTESIAN_POINT('Ctrl Pts',(-53.905727267535,-15.1159903036539,176.219573585739));
#15285=CARTESIAN_POINT('Ctrl Pts',(-53.6343010604909,-14.9449274325696,
177.258764585683));
#15286=CARTESIAN_POINT('Ctrl Pts',(-52.3195045847479,-14.4589334435455,
178.541768722646));
#15287=CARTESIAN_POINT('Ctrl Pts',(-51.3015568868895,-14.1438839803641,
178.764698457169));
#15288=CARTESIAN_POINT('Ctrl Pts',(-49.5920248617255,-13.5797433288121,
178.136857041975));
#15289=CARTESIAN_POINT('Ctrl Pts',(-48.9380275082558,-13.3381062047143,
177.30578604004));
#15290=CARTESIAN_POINT('Ctrl Pts',(-48.7105476579708,-13.0557925005452,
175.429441731563));
#15291=CARTESIAN_POINT('Ctrl Pts',(-49.1406103931943,-13.0235604552581,
174.438788862592));
#15292=CARTESIAN_POINT('Ctrl Pts',(-50.6761207099769,-13.0860799668151,
173.321489243126));
#15293=CARTESIAN_POINT('Ctrl Pts',(-51.7550963134731,-13.1754760058423,
173.222308149713));
#15294=CARTESIAN_POINT('Ctrl Pts',(-53.4658619993328,-13.2728668841322,
174.044907498799));
#15295=CARTESIAN_POINT('Ctrl Pts',(-54.0695830139971,-13.2704822339251,
174.951304580462));
#15296=CARTESIAN_POINT('Ctrl Pts',(-54.1756431350045,-13.0566118191168,
176.841599266944));
#15297=CARTESIAN_POINT('Ctrl Pts',(-53.682402379201,-12.8459201272062,177.784941606983));
#15298=CARTESIAN_POINT('Ctrl Pts',(-52.1086906323698,-12.3039548020853,
178.724742549594));
#15299=CARTESIAN_POINT('Ctrl Pts',(-51.0761365726385,-11.9897880340734,
178.697123202695));
#15300=CARTESIAN_POINT('Ctrl Pts',(-49.5543778605173,-11.4626036611189,
177.68675201361));
#15301=CARTESIAN_POINT('Ctrl Pts',(-49.102117382649,-11.2567014833508,176.719561205716));
#15302=CARTESIAN_POINT('Ctrl Pts',(-49.292107286816,-11.0609269687249,174.839303437302));
#15303=CARTESIAN_POINT('Ctrl Pts',(-49.9319808722111,-11.065488255827,173.957841233623));
#15304=CARTESIAN_POINT('Ctrl Pts',(-51.6826661337304,-11.1687038756892,
173.21175444078));
#15305=CARTESIAN_POINT('Ctrl Pts',(-52.7531972098707,-11.2596980870477,
173.357216390535));
#15306=CARTESIAN_POINT('Ctrl Pts',(-54.2460458385202,-11.3089418781751,
174.551734842451));
#15307=CARTESIAN_POINT('Ctrl Pts',(-54.6245671161656,-11.2668768405657,
175.56211463078));
#15308=CARTESIAN_POINT('Ctrl Pts',(-54.3123472668563,-10.9730441873765,
177.413426209709));
#15309=CARTESIAN_POINT('Ctrl Pts',(-53.6216949876352,-10.7211032153202,
178.215314744748));
#15310=CARTESIAN_POINT('Ctrl Pts',(-51.8913746121094,-10.1550133368813,
178.758899998487));
#15311=CARTESIAN_POINT('Ctrl Pts',(-50.8831280746124,-9.84182247697009,
178.493145848044));
#15312=CARTESIAN_POINT('Ctrl Pts',(-49.6236112332636,-9.36447275925141,
177.143870489208));
#15313=CARTESIAN_POINT('Ctrl Pts',(-49.3975849797945,-9.20540142615231,
176.095279478262));
#15314=CARTESIAN_POINT('Ctrl Pts',(-50.0079456983536,-9.08466255147406,
174.288405253537));
#15315=CARTESIAN_POINT('Ctrl Pts',(-50.8244602905949,-9.12692713822202,
173.581609594638));
#15316=CARTESIAN_POINT('Ctrl Pts',(-52.6906598209441,-9.25318698046637,
173.246687842459));
#15317=CARTESIAN_POINT('Ctrl Pts',(-53.7047460872083,-9.33006604421617,
173.631253257821));
#15318=CARTESIAN_POINT('Ctrl Pts',(-54.8900559939021,-9.32613298909108,
175.117109460381));
#15319=CARTESIAN_POINT('Ctrl Pts',(-55.0428852800419,-9.23680213120813,
176.191613835385));
#15320=CARTESIAN_POINT('Ctrl Pts',(-54.3260630027991,-8.86426623816917,
177.917066297754));
#15321=CARTESIAN_POINT('Ctrl Pts',(-53.4783261791472,-8.5852751826903,178.533414961083));
#15322=CARTESIAN_POINT('Ctrl Pts',(-51.6632029807945,-7.99669600625119,
178.652882987613));
#15323=CARTESIAN_POINT('Ctrl Pts',(-50.7499980781025,-7.70554604519678,
178.155739114359));
#15324=CARTESIAN_POINT('Ctrl Pts',(-49.8242259537338,-7.29327695933862,
176.547077701437));
#15325=CARTESIAN_POINT('Ctrl Pts',(-49.838033268214,-7.17726487827271,175.466032067978));
#15326=CARTESIAN_POINT('Ctrl Pts',(-50.8256764893838,-7.13523953214819,
173.842841571287));
#15327=CARTESIAN_POINT('Ctrl Pts',(-51.7828991970818,-7.20106754009712,
173.328393136411));
#15328=CARTESIAN_POINT('Ctrl Pts',(-53.682121466631,-7.33289296119618,173.423267613666));
#15329=CARTESIAN_POINT('Ctrl Pts',(-54.5824458512144,-7.39109185214275,
174.023927494841));
#15330=CARTESIAN_POINT('Ctrl Pts',(-55.4117106483233,-7.31244449093335,
175.744908515432));
#15331=CARTESIAN_POINT('Ctrl Pts',(-55.3174225063257,-7.17911919393448,
176.81298142285));
#15332=CARTESIAN_POINT('Ctrl Pts',(-54.241836216539,-6.73809069114013,178.316074643566));
#15333=CARTESIAN_POINT('Ctrl Pts',(-53.2777666803375,-6.43346338348791,
178.716995563853));
#15334=CARTESIAN_POINT('Ctrl Pts',(-51.492709987459,-5.85671796076922,178.410389321177));
#15335=CARTESIAN_POINT('Ctrl Pts',(-50.7047045568934,-5.58599179870949,
177.709705935534));
#15336=CARTESIAN_POINT('Ctrl Pts',(-50.1611589540997,-5.24690475917716,
175.91572047402));
#15337=CARTESIAN_POINT('Ctrl Pts',(-50.412988668319,-5.17989675417243,174.862537959116));
#15338=CARTESIAN_POINT('Ctrl Pts',(-51.7459369624996,-5.19848686371817,
173.493142781303));
#15339=CARTESIAN_POINT('Ctrl Pts',(-52.7859565461007,-5.28395186106844,
173.214419006065));
#15340=CARTESIAN_POINT('Ctrl Pts',(-54.6124153348595,-5.40237052054082,
173.730440016312));
#15341=CARTESIAN_POINT('Ctrl Pts',(-55.3590089692939,-5.42765093815174,
174.520747942326));
#15342=CARTESIAN_POINT('Ctrl Pts',(-55.7857743262001,-5.27753030569205,
176.366096056906));
#15343=CARTESIAN_POINT('Ctrl Pts',(-55.461398252989,-5.09617167994865,177.38970404608));
#15344=CARTESIAN_POINT('Ctrl Pts',(-54.0763289367501,-4.5947076574371,178.59887213214));
#15345=CARTESIAN_POINT('Ctrl Pts',(-53.0518069694618,-4.2817330879142,178.762764238352));
#15346=CARTESIAN_POINT('Ctrl Pts',(-51.3741810061549,-3.71961935803744,
178.037173193724));
#15347=CARTESIAN_POINT('Ctrl Pts',(-50.7709128345885,-3.48817293681553,
177.171361011829));
#15348=CARTESIAN_POINT('Ctrl Pts',(-50.6389382081356,-3.22905679794207,
175.293151941354));
#15349=CARTESIAN_POINT('Ctrl Pts',(-51.12053621277,-3.20321300476925,174.318272388974));
#15350=CARTESIAN_POINT('Ctrl Pts',(-52.7133196362096,-3.27785561089881,
173.283689189228));
#15351=CARTESIAN_POINT('Ctrl Pts',(-53.7973395798457,-3.36818712000785,
173.24106430149));
#15352=CARTESIAN_POINT('Ctrl Pts',(-55.4653436163453,-3.45546685002776,
174.15674387015));
#15353=CARTESIAN_POINT('Ctrl Pts',(-56.0173052873986,-3.44570666511222,
175.091057375796));
#15354=CARTESIAN_POINT('Ctrl Pts',(-56.0215539606611,-3.28449111210032,
176.384962205932));
#15355=CARTESIAN_POINT('Ctrl Pts',(-55.9545655524391,-3.23079314429921,
176.725242297786));
#15356=CARTESIAN_POINT('Ctrl Pts',(-55.7610730366685,-3.12770940060629,
177.200137919422));
#15357=CARTESIAN_POINT('Ctrl Pts',(-55.6813772878146,-3.09105284269064,
177.349953976371));
#15358=CARTESIAN_POINT('Ctrl Pts',(-55.542047034587,-3.0325075684579,177.559861392858));
#15359=CARTESIAN_POINT('Ctrl Pts',(-55.4922962422521,-3.01237854056411,
177.627368088468));
#15360=CARTESIAN_POINT('Ctrl Pts',(-55.3864710916189,-2.97076694703694,
177.757099244203));
#15361=CARTESIAN_POINT('Ctrl Pts',(-55.3343400650611,-2.9517036220202,177.814670571915));
#15362=CARTESIAN_POINT('Ctrl Pts',(-55.2712257966423,-2.92704897744562,
177.878689530232));
#15363=CARTESIAN_POINT('Ctrl Pts',(-50.193114320713,-27.8005016688432,177.448440461337));
#15364=CARTESIAN_POINT('Ctrl Pts',(-50.1356777281885,-27.7780416249781,
177.514251363723));
#15365=CARTESIAN_POINT('Ctrl Pts',(-50.0768656935625,-27.751543311514,177.569181845458));
#15366=CARTESIAN_POINT('Ctrl Pts',(-49.9502510673185,-27.7006718917524,
177.678131488152));
#15367=CARTESIAN_POINT('Ctrl Pts',(-49.8836384545372,-27.6746069642733,
177.728584647058));
#15368=CARTESIAN_POINT('Ctrl Pts',(-49.6751767137455,-27.5945945456976,
177.866776279515));
#15369=CARTESIAN_POINT('Ctrl Pts',(-49.5241175159801,-27.5384622401806,
177.941191651987));
#15370=CARTESIAN_POINT('Ctrl Pts',(-49.052722448706,-27.3677108924734,178.102046365205));
#15371=CARTESIAN_POINT('Ctrl Pts',(-48.713006227557,-27.2491092781452,178.126053652285));
#15372=CARTESIAN_POINT('Ctrl Pts',(-47.7382795874562,-26.9019657740439,
177.942209528285));
#15373=CARTESIAN_POINT('Ctrl Pts',(-47.1597470877608,-26.6842880122364,
177.461567693823));
#15374=CARTESIAN_POINT('Ctrl Pts',(-46.658904710499,-26.3725604903201,176.179580952166));
#15375=CARTESIAN_POINT('Ctrl Pts',(-46.744016732095,-26.2835354545934,175.410971277798));
#15376=CARTESIAN_POINT('Ctrl Pts',(-47.5354179070377,-26.2224078706935,
174.242909311213));
#15377=CARTESIAN_POINT('Ctrl Pts',(-48.2245449656354,-26.2493771368743,
173.87343933243));
#15378=CARTESIAN_POINT('Ctrl Pts',(-49.6317089464608,-26.3060463238627,
173.871895146128));
#15379=CARTESIAN_POINT('Ctrl Pts',(-50.3230600395606,-26.332977077053,174.238655026377));
#15380=CARTESIAN_POINT('Ctrl Pts',(-51.1153496063116,-26.2743348509258,
175.387691644257));
#15381=CARTESIAN_POINT('Ctrl Pts',(-51.2096393582444,-26.1855070701005,
176.164686974611));
#15382=CARTESIAN_POINT('Ctrl Pts',(-50.7213268039385,-25.8775623946772,
177.442968877094));
#15383=CARTESIAN_POINT('Ctrl Pts',(-50.1473617008829,-25.6602454668112,
177.932812658479));
#15384=CARTESIAN_POINT('Ctrl Pts',(-48.8451246534299,-25.1962898596545,
178.190564242377));
#15385=CARTESIAN_POINT('Ctrl Pts',(-48.1356293396501,-24.9529458243571,
177.955714348281));
#15386=CARTESIAN_POINT('Ctrl Pts',(-47.2268076672755,-24.5631416907191,
176.954286183848));
#15387=CARTESIAN_POINT('Ctrl Pts',(-47.0395646158613,-24.4209960169422,
176.20954077848));
#15388=CARTESIAN_POINT('Ctrl Pts',(-47.370313215787,-24.2726666068476,174.855768290097));
#15389=CARTESIAN_POINT('Ctrl Pts',(-47.8845545017147,-24.265674947158,174.26583855031));
#15390=CARTESIAN_POINT('Ctrl Pts',(-49.1994460468846,-24.3046603227726,
173.764180115318));
#15391=CARTESIAN_POINT('Ctrl Pts',(-49.9762257647407,-24.3480555327739,
173.861039734223));
#15392=CARTESIAN_POINT('Ctrl Pts',(-51.1285193941288,-24.3574791486806,
174.66646218052));
#15393=CARTESIAN_POINT('Ctrl Pts',(-51.4882290443068,-24.3203491702665,
175.364132112564));
#15394=CARTESIAN_POINT('Ctrl Pts',(-51.4777341832408,-24.1036300286494,
176.755680066459));
#15395=CARTESIAN_POINT('Ctrl Pts',(-51.1141102527119,-23.9275319100486,
177.423612084264));
#15396=CARTESIAN_POINT('Ctrl Pts',(-49.9940329966114,-23.4994535030053,
178.148719290634));
#15397=CARTESIAN_POINT('Ctrl Pts',(-49.2531996565364,-23.2503850964097,
178.195074921104));
#15398=CARTESIAN_POINT('Ctrl Pts',(-48.0540724826088,-22.804580182732,177.607487959387));
#15399=CARTESIAN_POINT('Ctrl Pts',(-47.6174629086983,-22.6140260251447,
176.985139741962));
#15400=CARTESIAN_POINT('Ctrl Pts',(-47.4549919432363,-22.3698803060775,
175.609945370482));
#15401=CARTESIAN_POINT('Ctrl Pts',(-47.7329522193418,-22.3169255939418,
174.876470615888));
#15402=CARTESIAN_POINT('Ctrl Pts',(-48.8440385240951,-22.3059754149369,
173.902867041218));
#15403=CARTESIAN_POINT('Ctrl Pts',(-49.7035599970344,-22.3554674780819,
173.739637329099));
#15404=CARTESIAN_POINT('Ctrl Pts',(-51.1531706356154,-22.4011313967338,
174.265066374312));
#15405=CARTESIAN_POINT('Ctrl Pts',(-51.7115054154064,-22.3910761212842,
174.945624054023));
#15406=CARTESIAN_POINT('Ctrl Pts',(-51.9563259347572,-22.2045289991918,
176.459132103654));
#15407=CARTESIAN_POINT('Ctrl Pts',(-51.63765119649,-22.0251559400258,177.262331468575));
#15408=CARTESIAN_POINT('Ctrl Pts',(-50.4571461815608,-21.5627984935069,
178.149907937338));
#15409=CARTESIAN_POINT('Ctrl Pts',(-49.6222512854117,-21.2849471395443,
178.217719280236));
#15410=CARTESIAN_POINT('Ctrl Pts',(-48.3256452005116,-20.7988977065915,
177.525255091295));
#15411=CARTESIAN_POINT('Ctrl Pts',(-47.8935170509031,-20.5993012814682,
176.78942555283));
#15412=CARTESIAN_POINT('Ctrl Pts',(-47.9069259765589,-20.3679964193449,
175.264267840625));
#15413=CARTESIAN_POINT('Ctrl Pts',(-48.3565963500671,-20.33698501403,174.508050023486));
#15414=CARTESIAN_POINT('Ctrl Pts',(-49.7115395236169,-20.3645147337819,
173.767258025586));
#15415=CARTESIAN_POINT('Ctrl Pts',(-50.5919963646361,-20.4163759449694,
173.798730113887));
#15416=CARTESIAN_POINT('Ctrl Pts',(-51.8921615926268,-20.4324111199544,
174.637786957993));
#15417=CARTESIAN_POINT('Ctrl Pts',(-52.2870845316673,-20.391715494119,175.425932171935));
#15418=CARTESIAN_POINT('Ctrl Pts',(-52.1845249551972,-20.1359343420921,
176.949348485014));
#15419=CARTESIAN_POINT('Ctrl Pts',(-51.6978717551623,-19.9258306519252,
177.647217385389));
#15420=CARTESIAN_POINT('Ctrl Pts',(-50.3567743114224,-19.4332812849397,
178.229888643815));
#15421=CARTESIAN_POINT('Ctrl Pts',(-49.531482093434,-19.1564117811874,178.098575810452));
#15422=CARTESIAN_POINT('Ctrl Pts',(-48.4209526978951,-18.7085233315365,
177.123331466978));
#15423=CARTESIAN_POINT('Ctrl Pts',(-48.1597795720535,-18.5402167412103,
176.29718764283));
#15424=CARTESIAN_POINT('Ctrl Pts',(-48.5145782694716,-18.3739619700934,
174.800216258582));
#15425=CARTESIAN_POINT('Ctrl Pts',(-49.1216168980297,-18.3741927637648,
174.159897255644));
#15426=CARTESIAN_POINT('Ctrl Pts',(-50.6124880467131,-18.4256628314289,
173.74530968569));
#15427=CARTESIAN_POINT('Ctrl Pts',(-51.4570089590119,-18.472296203581,173.973986288395));
#15428=CARTESIAN_POINT('Ctrl Pts',(-52.5367755134872,-18.4465314340497,
175.076321400051));
#15429=CARTESIAN_POINT('Ctrl Pts',(-52.7461464663159,-18.3691716102472,
175.928004990245));
#15430=CARTESIAN_POINT('Ctrl Pts',(-52.3166330239091,-18.0526500335514,
177.376965544067));
#15431=CARTESIAN_POINT('Ctrl Pts',(-51.6857211698905,-17.8130496454,177.945754508989));
#15432=CARTESIAN_POINT('Ctrl Pts',(-50.2465394893753,-17.3007990625156,
178.194297846636));
#15433=CARTESIAN_POINT('Ctrl Pts',(-49.4703000985441,-17.0343670318334,
177.871754882023));
#15434=CARTESIAN_POINT('Ctrl Pts',(-48.6088763818932,-16.6321365971318,
176.648991214725));
#15435=CARTESIAN_POINT('Ctrl Pts',(-48.5409020769561,-16.5028432711256,
175.78526591443));
#15436=CARTESIAN_POINT('Ctrl Pts',(-49.2164515058916,-16.3991203888251,
174.401518908745));
#15437=CARTESIAN_POINT('Ctrl Pts',(-49.9496118192587,-16.4227354715302,
173.914202886417));
#15438=CARTESIAN_POINT('Ctrl Pts',(-51.4902606534728,-16.4861638259448,
173.836744887307));
#15439=CARTESIAN_POINT('Ctrl Pts',(-52.2697075969923,-16.5185243960147,
174.249627738192));
#15440=CARTESIAN_POINT('Ctrl Pts',(-53.0792623986938,-16.4399376212412,
175.566241461313));
#15441=CARTESIAN_POINT('Ctrl Pts',(-53.0958608617722,-16.3264383488088,
176.440260240546));
#15442=CARTESIAN_POINT('Ctrl Pts',(-52.3498924896565,-15.9464100326616,
177.743856795072));
#15443=CARTESIAN_POINT('Ctrl Pts',(-51.6136771994172,-15.6882407493956,
178.142477224647));
#15444=CARTESIAN_POINT('Ctrl Pts',(-50.1619939854693,-15.1743526813971,
178.045393567771));
#15445=CARTESIAN_POINT('Ctrl Pts',(-49.479535393056,-14.9249532161513,177.547481856475));
#15446=CARTESIAN_POINT('Ctrl Pts',(-48.9083003859244,-14.5811172796918,
176.154888290848));
#15447=CARTESIAN_POINT('Ctrl Pts',(-49.032687325759,-14.4872017268269,175.286386043965));
#15448=CARTESIAN_POINT('Ctrl Pts',(-50.002899927607,-14.4395306566209,174.08106638639));
#15449=CARTESIAN_POINT('Ctrl Pts',(-50.8258619899905,-14.4815667576624,
173.768688449528));
#15450=CARTESIAN_POINT('Ctrl Pts',(-52.3490472247602,-14.5391579602322,
174.044477097964));
#15451=CARTESIAN_POINT('Ctrl Pts',(-53.0108480437211,-14.5505369630929,
174.618897762295));
#15452=CARTESIAN_POINT('Ctrl Pts',(-53.508606726061,-14.41258118913,176.072854784516));
#15453=CARTESIAN_POINT('Ctrl Pts',(-53.3308496256547,-14.2605010523332,
176.92211652172));
#15454=CARTESIAN_POINT('Ctrl Pts',(-52.3234046589676,-13.8325238003689,
178.011250192421));
#15455=CARTESIAN_POINT('Ctrl Pts',(-51.5138129382755,-13.5585438056648,
178.229366209696));
#15456=CARTESIAN_POINT('Ctrl Pts',(-50.1182607249297,-13.0546721198729,
177.788098654291));
#15457=CARTESIAN_POINT('Ctrl Pts',(-49.5630188185408,-12.8308644828691,
177.140857971114));
#15458=CARTESIAN_POINT('Ctrl Pts',(-49.3219040202974,-12.5483689245281,
175.637957478437));
#15459=CARTESIAN_POINT('Ctrl Pts',(-49.6365594730894,-12.4926951709364,
174.821179942866));
#15460=CARTESIAN_POINT('Ctrl Pts',(-50.8450351424658,-12.4918253386163,
173.862170041067));
#15461=CARTESIAN_POINT('Ctrl Pts',(-51.7160671936879,-12.5420406725331,
173.742988789581));
#15462=CARTESIAN_POINT('Ctrl Pts',(-53.1380531234061,-12.5824907099911,
174.344563971126));
#15463=CARTESIAN_POINT('Ctrl Pts',(-53.661497991413,-12.565516429584,175.054752397452));
#15464=CARTESIAN_POINT('Ctrl Pts',(-53.8242077932451,-12.3622912981454,
176.579637740953));
#15465=CARTESIAN_POINT('Ctrl Pts',(-53.4635573374974,-12.1759538811977,
177.362604506387));
#15466=CARTESIAN_POINT('Ctrl Pts',(-52.2358756182636,-11.7031645393402,
178.179207046235));
#15467=CARTESIAN_POINT('Ctrl Pts',(-51.404471480006,-11.4266005921062,178.198059647233));
#15468=CARTESIAN_POINT('Ctrl Pts',(-50.1465877134854,-10.9499764840513,
177.440684540534));
#15469=CARTESIAN_POINT('Ctrl Pts',(-49.7512566691313,-10.7559713173261,
176.677961727673));
#15470=CARTESIAN_POINT('Ctrl Pts',(-49.8442980389787,-10.5402489724976,
175.152069846099));
#15471=CARTESIAN_POINT('Ctrl Pts',(-50.3336227209985,-10.5166703329192,
174.417963751365));
#15472=CARTESIAN_POINT('Ctrl Pts',(-51.729412313951,-10.5511670115394,173.750914008412));
#15473=CARTESIAN_POINT('Ctrl Pts',(-52.6055357660183,-10.6034581645062,
173.829125569603));
#15474=CARTESIAN_POINT('Ctrl Pts',(-53.8591972775733,-10.6090268187652,
174.739479897504));
#15475=CARTESIAN_POINT('Ctrl Pts',(-54.2075655427863,-10.559958422732,175.542285446703));
#15476=CARTESIAN_POINT('Ctrl Pts',(-54.0309723767407,-10.2919570312328,
177.05153449857));
#15477=CARTESIAN_POINT('Ctrl Pts',(-53.5065211660476,-10.0729835636969,
177.724885949439));
#15478=CARTESIAN_POINT('Ctrl Pts',(-52.1359327706082,-9.57501150980407,
178.231990439602));
#15479=CARTESIAN_POINT('Ctrl Pts',(-51.3168725161042,-9.29919601638729,
178.055337178134));
#15480=CARTESIAN_POINT('Ctrl Pts',(-50.258716477129,-8.86039345968628,177.014257444883));
#15481=CARTESIAN_POINT('Ctrl Pts',(-50.0419858596938,-8.70190296068798,
176.174822144773));
#15482=CARTESIAN_POINT('Ctrl Pts',(-50.4788136762356,-8.55014763089762,
174.697436550109));
#15483=CARTESIAN_POINT('Ctrl Pts',(-51.1165600370436,-8.55674976323144,
174.095019459488));
#15484=CARTESIAN_POINT('Ctrl Pts',(-52.6206590619166,-8.6128620697194,173.755704628284));
#15485=CARTESIAN_POINT('Ctrl Pts',(-53.456626592603,-8.65630954771657,174.029197443714));
#15486=CARTESIAN_POINT('Ctrl Pts',(-54.4781193003427,-8.6195332279715,175.187078119489));
#15487=CARTESIAN_POINT('Ctrl Pts',(-54.643602443466,-8.53353572012608,176.04949882023));
#15488=CARTESIAN_POINT('Ctrl Pts',(-54.1354947853707,-8.20096498746117,
177.472181687833));
#15489=CARTESIAN_POINT('Ctrl Pts',(-53.4760203027823,-7.95706608118669,
178.003825172765));
#15490=CARTESIAN_POINT('Ctrl Pts',(-52.0249165538012,-7.441132564782,178.167825277993));
#15491=CARTESIAN_POINT('Ctrl Pts',(-51.2723007652614,-7.17976116760829,
177.802466009854));
#15492=CARTESIAN_POINT('Ctrl Pts',(-50.4742318046734,-6.79179686888332,
176.539214575509));
#15493=CARTESIAN_POINT('Ctrl Pts',(-50.4508393849021,-6.66952799804251,
175.667365550039));
#15494=CARTESIAN_POINT('Ctrl Pts',(-51.1982775200671,-6.57992894303025,
174.318931761547));
#15495=CARTESIAN_POINT('Ctrl Pts',(-51.9567203354133,-6.60831910752051,
173.869388776842));
#15496=CARTESIAN_POINT('Ctrl Pts',(-53.5030461170827,-6.67180659392302,
173.876188814802));
#15497=CARTESIAN_POINT('Ctrl Pts',(-54.2579318048227,-6.70074853854407,
174.329266762268));
#15498=CARTESIAN_POINT('Ctrl Pts',(-54.9950541895712,-6.6067812144727,175.688231083653));
#15499=CARTESIAN_POINT('Ctrl Pts',(-54.9633937640365,-6.48434226598442,
176.556150922255));
#15500=CARTESIAN_POINT('Ctrl Pts',(-54.1573516980127,-6.0949735677162,177.812809342709));
#15501=CARTESIAN_POINT('Ctrl Pts',(-53.3979887985791,-5.83073710308303,
178.172806822259));
#15502=CARTESIAN_POINT('Ctrl Pts',(-51.9519097716579,-5.31810666795101,
177.994568269632));
#15503=CARTESIAN_POINT('Ctrl Pts',(-51.2952074816856,-5.0735953089356,177.458800517348));
#15504=CARTESIAN_POINT('Ctrl Pts',(-50.7993635736617,-4.74342220821161,
176.031468409862));
#15505=CARTESIAN_POINT('Ctrl Pts',(-50.9692613848378,-4.65940397939939,
175.170313217647));
#15506=CARTESIAN_POINT('Ctrl Pts',(-52.0040245669764,-4.62293999106357,
174.01934301833));
#15507=CARTESIAN_POINT('Ctrl Pts',(-52.8385688131003,-4.66759138415716,
173.754231358386));
#15508=CARTESIAN_POINT('Ctrl Pts',(-54.3414847379305,-4.72329909029368,
174.103969484305));
#15509=CARTESIAN_POINT('Ctrl Pts',(-54.9761466933045,-4.72791014175074,
174.714716972292));
#15510=CARTESIAN_POINT('Ctrl Pts',(-55.3975165431988,-4.57549651155636,
176.192173272167));
#15511=CARTESIAN_POINT('Ctrl Pts',(-55.1760506072609,-4.4148786220368,177.03103539143));
#15512=CARTESIAN_POINT('Ctrl Pts',(-54.1093043232961,-3.97451188101218,
178.061753391873));
#15513=CARTESIAN_POINT('Ctrl Pts',(-53.2902925544343,-3.69995792969149,
178.233822626392));
#15514=CARTESIAN_POINT('Ctrl Pts',(-51.9203920380846,-3.19963469730891,
177.711493690972));
#15515=CARTESIAN_POINT('Ctrl Pts',(-51.4044324721558,-2.98383265912278,
177.036002564632));
#15516=CARTESIAN_POINT('Ctrl Pts',(-51.237949425703,-2.71774512370317,175.525044339462));
#15517=CARTESIAN_POINT('Ctrl Pts',(-51.5957499271559,-2.66894330374766,
174.721509320474));
#15518=CARTESIAN_POINT('Ctrl Pts',(-52.8541051305037,-2.67783999801612,
173.825937213487));
#15519=CARTESIAN_POINT('Ctrl Pts',(-53.7315999697276,-2.7292086653859,173.7525048498));
#15520=CARTESIAN_POINT('Ctrl Pts',(-55.1208667949195,-2.76252327401043,
174.431246184642));
#15521=CARTESIAN_POINT('Ctrl Pts',(-55.6054709668258,-2.73893798071373,
175.167402226862));
#15522=CARTESIAN_POINT('Ctrl Pts',(-55.6603171863937,-2.58869274068622,
176.211840888345));
#15523=CARTESIAN_POINT('Ctrl Pts',(-55.6210463302226,-2.5392081864434,176.490448482462));
#15524=CARTESIAN_POINT('Ctrl Pts',(-55.4836397365907,-2.4479441182576,176.880586390838));
#15525=CARTESIAN_POINT('Ctrl Pts',(-55.4253285390117,-2.41535251334816,
177.005027857449));
#15526=CARTESIAN_POINT('Ctrl Pts',(-55.321414213033,-2.36345060131236,177.180440236558));
#15527=CARTESIAN_POINT('Ctrl Pts',(-55.2840225057543,-2.34563722905757,
177.23703696138));
#15528=CARTESIAN_POINT('Ctrl Pts',(-55.2039936793606,-2.30896761153951,
177.345998347345));
#15529=CARTESIAN_POINT('Ctrl Pts',(-55.1587206712145,-2.28906361698866,
177.401367187303));
#15530=CARTESIAN_POINT('Ctrl Pts',(-55.1161897096451,-2.27071607222657,
177.448351373365));
#15531=CARTESIAN_POINT('Origin',(-49.8994188116831,-27.9943596339097,177.258277275215));
#15532=CARTESIAN_POINT('Ctrl Pts',(-47.8886718415116,-31.6995536639001,
175.585485069079));
#15533=CARTESIAN_POINT('Ctrl Pts',(-47.9424090991571,-31.4208895534118,
175.585485069079));
#15534=CARTESIAN_POINT('Ctrl Pts',(-48.0165136638412,-31.142217631488,175.587595470504));
#15535=CARTESIAN_POINT('Ctrl Pts',(-48.206190379979,-30.6092681473582,175.5992945923));
#15536=CARTESIAN_POINT('Ctrl Pts',(-48.3219855416571,-30.3543443720961,
175.608895409754));
#15537=CARTESIAN_POINT('Ctrl Pts',(-48.7193595355016,-29.6463117438825,
175.654781597023));
#15538=CARTESIAN_POINT('Ctrl Pts',(-49.0545911241397,-29.252967076522,175.707428551708));
#15539=CARTESIAN_POINT('Ctrl Pts',(-49.5445318563166,-28.7861739714513,
175.852028081795));
#15540=CARTESIAN_POINT('Ctrl Pts',(-49.6987397911889,-28.6436248452838,
175.911397856293));
#15541=CARTESIAN_POINT('Ctrl Pts',(-49.9262155871255,-28.4691236019893,
176.025260422827));
#15542=CARTESIAN_POINT('Ctrl Pts',(-50.0186861454797,-28.4371266816906,
176.06691518842));
#15543=CARTESIAN_POINT('Ctrl Pts',(-50.1842299781189,-28.3689363752761,
176.173317219728));
#15544=CARTESIAN_POINT('Ctrl Pts',(-50.2569026354171,-28.3307458842207,
176.235836425973));
#15545=CARTESIAN_POINT('Ctrl Pts',(-50.4390882192945,-28.20291241382,176.455121758264));
#15546=CARTESIAN_POINT('Ctrl Pts',(-50.5079392950738,-28.0960057551614,
176.657103040121));
#15547=CARTESIAN_POINT('Ctrl Pts',(-50.4672993044493,-27.9634501974094,
176.968869644582));
#15548=CARTESIAN_POINT('Ctrl Pts',(-50.4326818607288,-27.9245995634275,
177.070967051899));
#15549=CARTESIAN_POINT('Ctrl Pts',(-50.3339110252539,-27.8569369682875,
177.264936028611));
#15550=CARTESIAN_POINT('Ctrl Pts',(-50.2683927599471,-27.8299386004748,
177.362186354007));
#15551=CARTESIAN_POINT('Ctrl Pts',(-50.193114320713,-27.8005016688432,177.448440461337));
#15552=CARTESIAN_POINT('Ctrl Pts',(-47.1031441589869,-31.5480734342088,
175.585485069079));
#15553=CARTESIAN_POINT('Ctrl Pts',(-47.1603662041614,-31.2513383379729,
175.585485069079));
#15554=CARTESIAN_POINT('Ctrl Pts',(-47.2482359974308,-30.9149655772776,
175.587875715227));
#15555=CARTESIAN_POINT('Ctrl Pts',(-47.4670950242505,-30.3000308864083,
175.601419934118));
#15556=CARTESIAN_POINT('Ctrl Pts',(-47.6018961077871,-30.0028542362142,
175.612574303893));
#15557=CARTESIAN_POINT('Ctrl Pts',(-48.06625584225,-29.1754899206181,175.666311941427));
#15558=CARTESIAN_POINT('Ctrl Pts',(-48.4618683742085,-28.7136853353929,
175.729732505271));
#15559=CARTESIAN_POINT('Ctrl Pts',(-49.0063756293611,-28.1949480459011,
175.890763292055));
#15560=CARTESIAN_POINT('Ctrl Pts',(-49.1677731230246,-28.0480163131157,
175.972468320302));
#15561=CARTESIAN_POINT('Ctrl Pts',(-49.3965343491423,-27.8703147335455,
176.056354650694));
#15562=CARTESIAN_POINT('Ctrl Pts',(-49.5042735598544,-27.8224509492496,
176.029622920355));
#15563=CARTESIAN_POINT('Ctrl Pts',(-49.714154138436,-27.7365778903946,176.021696276872));
#15564=CARTESIAN_POINT('Ctrl Pts',(-49.8092250008766,-27.6958009021663,
176.040400247712));
#15565=CARTESIAN_POINT('Ctrl Pts',(-50.0526599599857,-27.5670382667944,
176.149507116298));
#15566=CARTESIAN_POINT('Ctrl Pts',(-50.1573360552302,-27.4697774585579,
176.29868387691));
#15567=CARTESIAN_POINT('Ctrl Pts',(-50.1883082447542,-27.3362137867349,
176.557013250615));
#15568=CARTESIAN_POINT('Ctrl Pts',(-50.1794299894878,-27.2944646349798,
176.647304730812));
#15569=CARTESIAN_POINT('Ctrl Pts',(-50.1311335533471,-27.2163290407286,
176.829965813571));
#15570=CARTESIAN_POINT('Ctrl Pts',(-50.0905156624001,-27.1753600677279,
176.937389673553));
#15571=CARTESIAN_POINT('Ctrl Pts',(-50.0383214665825,-27.1440081492037,
177.018259765604));
#15572=CARTESIAN_POINT('Ctrl Pts',(-47.1031441589869,-31.5480734342088,
176.385485069079));
#15573=CARTESIAN_POINT('Ctrl Pts',(-47.1599854936771,-31.2533125799253,
176.385485069079));
#15574=CARTESIAN_POINT('Ctrl Pts',(-47.2462550636215,-30.9240508319461,
176.387855155919));
#15575=CARTESIAN_POINT('Ctrl Pts',(-47.460249087206,-30.3229192382893,176.401096636113));
#15576=CARTESIAN_POINT('Ctrl Pts',(-47.5913742255291,-30.0344018731676,
176.411980487031));
#15577=CARTESIAN_POINT('Ctrl Pts',(-48.0375122982338,-29.2397387684011,
176.463601555155));
#15578=CARTESIAN_POINT('Ctrl Pts',(-48.4124469809922,-28.8074108937189,
176.525602813253));
#15579=CARTESIAN_POINT('Ctrl Pts',(-48.8848496853331,-28.3577893519108,
176.665278154737));
#15580=CARTESIAN_POINT('Ctrl Pts',(-49.026848150992,-28.2513597906944,176.736022770841));
#15581=CARTESIAN_POINT('Ctrl Pts',(-49.1705854582322,-28.1079648662814,
176.786782875481));
#15582=CARTESIAN_POINT('Ctrl Pts',(-49.2060240792629,-28.0278386987345,
176.747088553392));
#15583=CARTESIAN_POINT('Ctrl Pts',(-49.2810889004422,-27.9003322593211,
176.67860791329));
#15584=CARTESIAN_POINT('Ctrl Pts',(-49.3144205003265,-27.8541778608178,
176.654181717029));
#15585=CARTESIAN_POINT('Ctrl Pts',(-49.3895778283813,-27.7529515714288,
176.588058724708));
#15586=CARTESIAN_POINT('Ctrl Pts',(-49.4143850760995,-27.7397337398683,
176.533088088996));
#15587=CARTESIAN_POINT('Ctrl Pts',(-49.4653959512805,-27.6892053509014,
176.504625861351));
#15588=CARTESIAN_POINT('Ctrl Pts',(-49.480846052191,-27.6666966453102,176.508814220202));
#15589=CARTESIAN_POINT('Ctrl Pts',(-49.4871117159947,-27.6078471194517,
176.551208753368));
#15590=CARTESIAN_POINT('Ctrl Pts',(-49.4794905861727,-27.5632681966532,
176.593760604048));
#15591=CARTESIAN_POINT('Ctrl Pts',(-49.4509304485228,-27.5317240793367,
176.63793339336));
#15592=CARTESIAN_POINT('Ctrl Pts',(-47.8886718415116,-31.6995536639001,
176.385485069079));
#15593=CARTESIAN_POINT('Ctrl Pts',(-47.9420283886728,-31.4228637953642,
176.385485069079));
#15594=CARTESIAN_POINT('Ctrl Pts',(-48.014532730032,-31.1513028861565,176.387574911196));
#15595=CARTESIAN_POINT('Ctrl Pts',(-48.1993444429345,-30.6321564992392,
176.398971294295));
#15596=CARTESIAN_POINT('Ctrl Pts',(-48.3114636593991,-30.3858920090494,
176.408301592892));
#15597=CARTESIAN_POINT('Ctrl Pts',(-48.6906159914853,-29.7105605916654,
176.452071210751));
#15598=CARTESIAN_POINT('Ctrl Pts',(-49.0051697309234,-29.3466926348484,
176.50329885969));
#15599=CARTESIAN_POINT('Ctrl Pts',(-49.4230059122887,-28.9490152774608,
176.626542944478));
#15600=CARTESIAN_POINT('Ctrl Pts',(-49.5578148191563,-28.8469683228627,
176.674952306832));
#15601=CARTESIAN_POINT('Ctrl Pts',(-49.7002666962155,-28.7067737347251,
176.755688647613));
#15602=CARTESIAN_POINT('Ctrl Pts',(-49.7204366648883,-28.6425144311754,
176.784380821457));
#15603=CARTESIAN_POINT('Ctrl Pts',(-49.7511647401251,-28.5326907442027,
176.830228856146));
#15604=CARTESIAN_POINT('Ctrl Pts',(-49.7620981348669,-28.4891228428723,
176.849617895289));
#15605=CARTESIAN_POINT('Ctrl Pts',(-49.7760060876902,-28.3888257184543,
176.893673366674));
#15606=CARTESIAN_POINT('Ctrl Pts',(-49.764988315943,-28.3659620364717,176.891507252207));
#15607=CARTESIAN_POINT('Ctrl Pts',(-49.7443870109756,-28.3164417615759,
176.916482255318));
#15608=CARTESIAN_POINT('Ctrl Pts',(-49.7340979234319,-28.2968315737579,
176.932476541289));
#15609=CARTESIAN_POINT('Ctrl Pts',(-49.6898891879014,-28.2484550470107,
176.986178968408));
#15610=CARTESIAN_POINT('Ctrl Pts',(-49.6573676837196,-28.2178467294001,
177.018557284502));
#15611=CARTESIAN_POINT('Ctrl Pts',(-49.6057233026532,-28.1882175989763,
177.068114089093));
#15612=CARTESIAN_POINT('Ctrl Pts',(-48.6741995240363,-31.8510338935913,
176.385485069079));
#15613=CARTESIAN_POINT('Ctrl Pts',(-48.7240712836685,-31.5924150108031,
176.385485069079));
#15614=CARTESIAN_POINT('Ctrl Pts',(-48.7828103964424,-31.3785549403669,
176.387294666473));
#15615=CARTESIAN_POINT('Ctrl Pts',(-48.9384397986629,-30.941393760189,176.396845952478));
#15616=CARTESIAN_POINT('Ctrl Pts',(-49.0315530932691,-30.7373821449313,
176.404622698753));
#15617=CARTESIAN_POINT('Ctrl Pts',(-49.3437196847369,-30.1813824149298,
176.440540866346));
#15618=CARTESIAN_POINT('Ctrl Pts',(-49.5978924808545,-29.8859743759779,
176.480994906127));
#15619=CARTESIAN_POINT('Ctrl Pts',(-49.9611621392443,-29.5402412030108,
176.587807734218));
#15620=CARTESIAN_POINT('Ctrl Pts',(-50.0887814873205,-29.442576855031,176.613881842823));
#15621=CARTESIAN_POINT('Ctrl Pts',(-50.2299479341988,-29.3055826031689,
176.724594419746));
#15622=CARTESIAN_POINT('Ctrl Pts',(-50.2348492505137,-29.2571901636164,
176.821673089522));
#15623=CARTESIAN_POINT('Ctrl Pts',(-50.221240579808,-29.1650492290843,176.981849799003));
#15624=CARTESIAN_POINT('Ctrl Pts',(-50.2097757694073,-29.1240678249268,
177.04505407355));
#15625=CARTESIAN_POINT('Ctrl Pts',(-50.162434346999,-29.0246998654798,177.199288008639));
#15626=CARTESIAN_POINT('Ctrl Pts',(-50.1155915557866,-28.9921903330752,
177.249926415417));
#15627=CARTESIAN_POINT('Ctrl Pts',(-50.0233780706706,-28.9436781722504,
177.328338649285));
#15628=CARTESIAN_POINT('Ctrl Pts',(-49.9873497946729,-28.9269665022055,
177.356138862376));
#15629=CARTESIAN_POINT('Ctrl Pts',(-49.8926666598081,-28.8890629745697,
177.421149183448));
#15630=CARTESIAN_POINT('Ctrl Pts',(-49.8352447812666,-28.872425262147,177.443353964955));
#15631=CARTESIAN_POINT('Ctrl Pts',(-49.7605161567837,-28.8447111186158,
177.498294784826));
#15632=CARTESIAN_POINT('Ctrl Pts',(-48.6741995240363,-31.8510338935913,
175.585485069079));
#15633=CARTESIAN_POINT('Ctrl Pts',(-48.7244519941528,-31.5904407688506,
175.585485069079));
#15634=CARTESIAN_POINT('Ctrl Pts',(-48.7847913302516,-31.3694696856984,
175.587315225781));
#15635=CARTESIAN_POINT('Ctrl Pts',(-48.9452857357075,-30.918505408308,175.597169250483));
#15636=CARTESIAN_POINT('Ctrl Pts',(-49.042074975527,-30.7058345079779,175.605216515615));
#15637=CARTESIAN_POINT('Ctrl Pts',(-49.3724632287533,-30.1171335671469,
175.643251252618));
#15638=CARTESIAN_POINT('Ctrl Pts',(-49.6473138740709,-29.7922488176511,
175.685124598145));
#15639=CARTESIAN_POINT('Ctrl Pts',(-50.0826880832722,-29.3773998970014,
175.813292871536));
#15640=CARTESIAN_POINT('Ctrl Pts',(-50.2297064593532,-29.239233377452,175.850327392284));
#15641=CARTESIAN_POINT('Ctrl Pts',(-50.4558968251088,-29.0679324704331,
175.99416619496));
#15642=CARTESIAN_POINT('Ctrl Pts',(-50.5330987311051,-29.0518024141316,
176.104207456485));
#15643=CARTESIAN_POINT('Ctrl Pts',(-50.6543058178018,-29.0012948601576,
176.324938162585));
#15644=CARTESIAN_POINT('Ctrl Pts',(-50.7045802699575,-28.9656908662752,
176.431272604233));
#15645=CARTESIAN_POINT('Ctrl Pts',(-50.8255164786033,-28.8387865608456,
176.760736400229));
#15646=CARTESIAN_POINT('Ctrl Pts',(-50.8585425349173,-28.722234051765,177.015522203332));
#15647=CARTESIAN_POINT('Ctrl Pts',(-50.7462903641443,-28.5906866080838,
177.38072603855));
#15648=CARTESIAN_POINT('Ctrl Pts',(-50.6859337319697,-28.5547344918753,
177.494629372986));
#15649=CARTESIAN_POINT('Ctrl Pts',(-50.5366884971606,-28.4975448958465,
177.699906243651));
#15650=CARTESIAN_POINT('Ctrl Pts',(-50.446269857494,-28.4845171332217,177.786983034461));
#15651=CARTESIAN_POINT('Ctrl Pts',(-50.3479071748434,-28.4569951884828,
177.87862115707));
#15652=CARTESIAN_POINT('Ctrl Pts',(-47.8886718415116,-31.6995536639001,
175.585485069079));
#15653=CARTESIAN_POINT('Ctrl Pts',(-47.9424090991571,-31.4208895534118,
175.585485069079));
#15654=CARTESIAN_POINT('Ctrl Pts',(-48.0165136638412,-31.142217631488,175.587595470504));
#15655=CARTESIAN_POINT('Ctrl Pts',(-48.206190379979,-30.6092681473582,175.5992945923));
#15656=CARTESIAN_POINT('Ctrl Pts',(-48.3219855416571,-30.3543443720961,
175.608895409754));
#15657=CARTESIAN_POINT('Ctrl Pts',(-48.7193595355016,-29.6463117438825,
175.654781597023));
#15658=CARTESIAN_POINT('Ctrl Pts',(-49.0545911241397,-29.252967076522,175.707428551708));
#15659=CARTESIAN_POINT('Ctrl Pts',(-49.5445318563166,-28.7861739714513,
175.852028081795));
#15660=CARTESIAN_POINT('Ctrl Pts',(-49.6987397911889,-28.6436248452838,
175.911397856293));
#15661=CARTESIAN_POINT('Ctrl Pts',(-49.9262155871255,-28.4691236019893,
176.025260422827));
#15662=CARTESIAN_POINT('Ctrl Pts',(-50.0186861454797,-28.4371266816906,
176.06691518842));
#15663=CARTESIAN_POINT('Ctrl Pts',(-50.1842299781189,-28.3689363752761,
176.173317219728));
#15664=CARTESIAN_POINT('Ctrl Pts',(-50.2569026354171,-28.3307458842207,
176.235836425973));
#15665=CARTESIAN_POINT('Ctrl Pts',(-50.4390882192945,-28.20291241382,176.455121758264));
#15666=CARTESIAN_POINT('Ctrl Pts',(-50.5079392950738,-28.0960057551614,
176.657103040121));
#15667=CARTESIAN_POINT('Ctrl Pts',(-50.4672993044493,-27.9634501974094,
176.968869644582));
#15668=CARTESIAN_POINT('Ctrl Pts',(-50.4326818607288,-27.9245995634275,
177.070967051899));
#15669=CARTESIAN_POINT('Ctrl Pts',(-50.3339110252539,-27.8569369682875,
177.264936028611));
#15670=CARTESIAN_POINT('Ctrl Pts',(-50.2683927599471,-27.8299386004748,
177.362186354007));
#15671=CARTESIAN_POINT('Ctrl Pts',(-50.193114320713,-27.8005016688432,177.448440461337));
#15672=CARTESIAN_POINT('Origin',(-54.5589537515075,2.89037996126418,174.712692862944));
#15673=CARTESIAN_POINT('Origin',(-47.4705283379689,-33.8679111978839,177.258277275215));
#47692=UNCERTAINTY_MEASURE_WITH_UNIT(LENGTH_MEASURE(0.01),#47718,
'DISTANCE_ACCURACY_VALUE',
'Maximum model space distance between geometric entities at asserted c
onnectivities');
#47703=UNCERTAINTY_MEASURE_WITH_UNIT(LENGTH_MEASURE(0.01),#47718,
'DISTANCE_ACCURACY_VALUE',
'Maximum model space distance between geometric entities at asserted c
onnectivities');
#47706=(
GEOMETRIC_REPRESENTATION_CONTEXT(3)
GLOBAL_UNCERTAINTY_ASSIGNED_CONTEXT((#47692))
GLOBAL_UNIT_ASSIGNED_CONTEXT((#47718,#47720,#47721))
REPRESENTATION_CONTEXT('','3D')
);
#47717=(
GEOMETRIC_REPRESENTATION_CONTEXT(3)
GLOBAL_UNCERTAINTY_ASSIGNED_CONTEXT((#47703))
GLOBAL_UNIT_ASSIGNED_CONTEXT((#47718,#47720,#47721))
REPRESENTATION_CONTEXT('','3D')
);
#47718=(
LENGTH_UNIT()
NAMED_UNIT(*)
SI_UNIT(.MILLI.,.METRE.)
);
#47720=(
NAMED_UNIT(*)
PLANE_ANGLE_UNIT()
SI_UNIT($,.RADIAN.)
);
#47721=(
NAMED_UNIT(*)
SI_UNIT($,.STERADIAN.)
SOLID_ANGLE_UNIT()
);
#47724=SHAPE_DEFINITION_REPRESENTATION(#47737,#47762);
#47737=PRODUCT_DEFINITION_SHAPE('',$,#47776);
#47762=SHAPE_REPRESENTATION('',(#9081),#47706);
#47773=PRODUCT_DEFINITION_CONTEXT('part definition',#47814,'design');
#47776=PRODUCT_DEFINITION('Tension Spring','Tension Spring',#47789,#47773);
#47789=PRODUCT_DEFINITION_FORMATION('',$,#47818);
#47814=APPLICATION_CONTEXT(
'Core Data for Automotive Mechanical Design Process');
#47815=PRODUCT_CONTEXT('part definition',#47814,'mechanical');
#47818=PRODUCT('Tension Spring','Tension Spring',$,(#47815));
#47830=PRESENTATION_STYLE_ASSIGNMENT((#47832));
#47832=SURFACE_STYLE_USAGE(.BOTH.,#47834);
#47834=SURFACE_SIDE_STYLE('',(#47836));
#47836=SURFACE_STYLE_FILL_AREA(#47838);
#47838=FILL_AREA_STYLE('Opaque(202,209,238)',(#47840));
#47840=FILL_AREA_STYLE_COLOUR('Opaque(202,209,238)',#47842);
#47842=COLOUR_RGB('Opaque(202,209,238)', 0.66274510, 0.83137255, 0.94901961);
ENDSEC;
END-ISO-10303-21;
